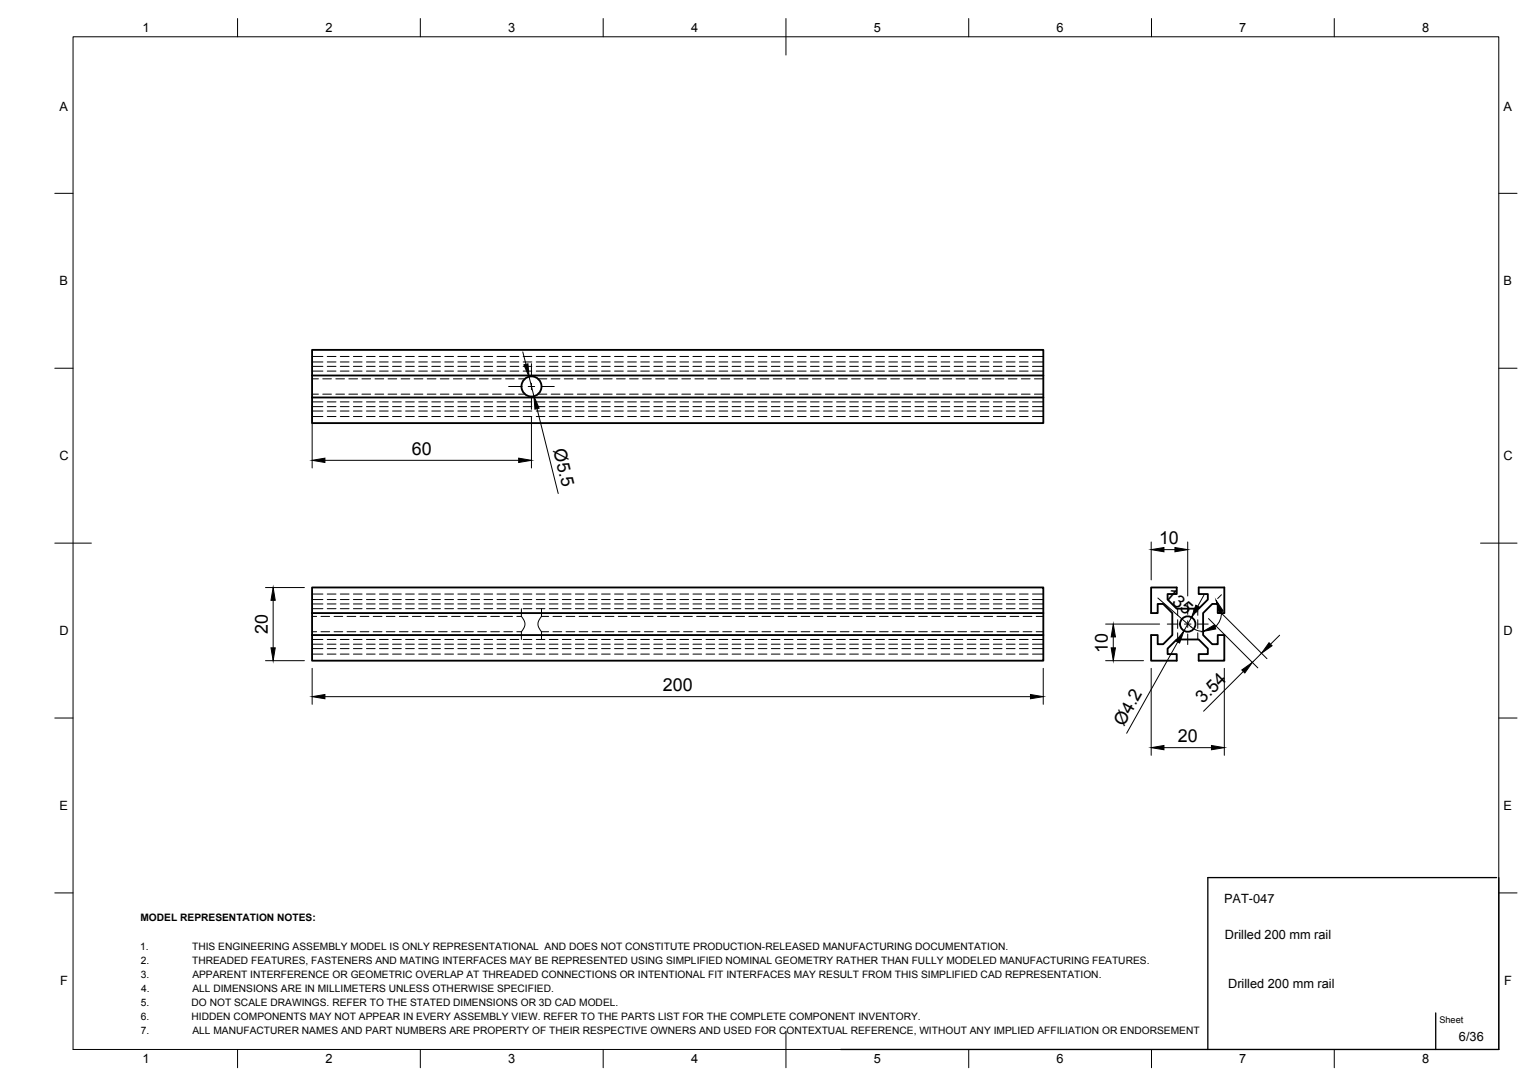
ISO-10303-21;
HEADER;
/* Generated by software containing ST-Developer
 * from STEP Tools, Inc. (www.steptools.com) 
 */

FILE_DESCRIPTION(
/* description */ ('Gravity roller conveyor section'),
/* implementation_level */ '2;1');

FILE_NAME(
/* name */ 'Drilled 200 mm rail.step',
/* time_stamp */ '2026-11-02T07:43:02-08:00',
/* author */ (''),
/* organization */ (''),
/* preprocessor_version */ 'ST-DEVELOPER v20.2',
/* originating_system */ 'Autodesk Translation Framework v15.17.0.0',
/* authorisation */ '');

FILE_SCHEMA (('AUTOMOTIVE_DESIGN { 1 0 10303 214 3 1 1 }'));
ENDSEC;

DATA;
#10=MECHANICAL_DESIGN_GEOMETRIC_PRESENTATION_REPRESENTATION('',(#531),#13821);
#438=B_SPLINE_CURVE_WITH_KNOTS('',3,(#11510,#11511,#11512,#11513,#11514,
#11515,#11516,#11517,#11518,#11519,#11520,#11521,#11522,#11523,#11524,#11525,
#11526,#11527,#11528,#11529,#11530,#11531),.UNSPECIFIED.,.F.,.F.,(4,2,2,
2,2,2,2,2,2,2,4),(0.335938049981195,0.418928967949028,0.501919885916861,
0.586897992939625,0.629387046451008,0.67187609996239,0.714365153473772,
0.756854206985154,0.841832314007919,0.924823231975752,1.00781414994358),
 .UNSPECIFIED.);
#439=B_SPLINE_CURVE_WITH_KNOTS('',3,(#11536,#11537,#11538,#11539,#11540,
#11541,#11542,#11543,#11544,#11545,#11546,#11547),.UNSPECIFIED.,.F.,.F.,
(4,2,2,2,2,4),(0.,0.0424890535113822,0.0849781070227644,0.169956214045529,
0.252947132013362,0.335938049981195),.UNSPECIFIED.);
#440=B_SPLINE_CURVE_WITH_KNOTS('',3,(#11548,#11549,#11550,#11551,#11552,
#11553,#11554,#11555,#11556,#11557,#11558,#11559),.UNSPECIFIED.,.F.,.F.,
(4,2,2,2,2,4),(1.00781414994358,1.09080506791142,1.17379598587925,1.25877409290202,
1.3012631464134,1.34375219992478),.UNSPECIFIED.);
#441=B_SPLINE_CURVE_WITH_KNOTS('',3,(#11562,#11563,#11564,#11565,#11566,
#11567,#11568,#11569,#11570,#11571,#11572,#11573,#11574,#11575,#11576,#11577,
#11578,#11579,#11580,#11581,#11582,#11583,#11584,#11585,#11586,#11587,#11588,
#11589,#11590,#11591,#11592,#11593),.UNSPECIFIED.,.F.,.F.,(4,2,2,2,2,2,
2,2,2,2,2,2,2,2,2,4),(0.,0.0424890535113822,0.0849781070227644,0.169956214045529,
0.252947132013362,0.335938049981195,0.418928967949028,0.501919885916861,
0.586897992939625,0.629387046451008,0.67187609996239,0.714365153473772,
0.756854206985154,0.841832314007919,0.924823231975752,1.00781414994358),
 .UNSPECIFIED.);
#442=B_SPLINE_CURVE_WITH_KNOTS('',3,(#11594,#11595,#11596,#11597,#11598,
#11599,#11600,#11601,#11602,#11603,#11604,#11605),.UNSPECIFIED.,.F.,.F.,
(4,2,2,2,2,4),(1.00781414994358,1.09080506791142,1.17379598587925,1.25877409290202,
1.3012631464134,1.34375219992478),.UNSPECIFIED.);
#463=SHAPE_REPRESENTATION_RELATIONSHIP('SRR','None',#14000,#497);
#497=ADVANCED_BREP_SHAPE_REPRESENTATION('',(#573),#13787);
#531=STYLED_ITEM('',(#14191),#573);
#573=MANIFOLD_SOLID_BREP('Body1',#7629);
#622=FACE_BOUND('',#1499,.T.);
#623=FACE_BOUND('',#1515,.T.);
#624=FACE_BOUND('',#1534,.T.);
#625=FACE_BOUND('',#1549,.T.);
#626=FACE_BOUND('',#1551,.T.);
#754=PLANE('',#8129);
#755=PLANE('',#8130);
#756=PLANE('',#8131);
#757=PLANE('',#8132);
#758=PLANE('',#8133);
#759=PLANE('',#8134);
#760=PLANE('',#8135);
#761=PLANE('',#8136);
#762=PLANE('',#8137);
#763=PLANE('',#8138);
#764=PLANE('',#8139);
#765=PLANE('',#8140);
#766=PLANE('',#8141);
#767=PLANE('',#8142);
#768=PLANE('',#8143);
#769=PLANE('',#8144);
#770=PLANE('',#8145);
#771=PLANE('',#8146);
#772=PLANE('',#8147);
#773=PLANE('',#8148);
#774=PLANE('',#8149);
#775=PLANE('',#8150);
#776=PLANE('',#8151);
#777=PLANE('',#8152);
#778=PLANE('',#8153);
#779=PLANE('',#8154);
#780=PLANE('',#8155);
#781=PLANE('',#8156);
#782=PLANE('',#8157);
#783=PLANE('',#8158);
#784=PLANE('',#8159);
#785=PLANE('',#8160);
#786=PLANE('',#8161);
#787=PLANE('',#8162);
#788=PLANE('',#8163);
#789=PLANE('',#8164);
#790=PLANE('',#8167);
#791=PLANE('',#8168);
#792=PLANE('',#8169);
#793=PLANE('',#8170);
#794=PLANE('',#8171);
#795=PLANE('',#8172);
#796=PLANE('',#8173);
#797=PLANE('',#8174);
#798=PLANE('',#8175);
#799=PLANE('',#8176);
#1066=FACE_OUTER_BOUND('',#1498,.T.);
#1067=FACE_OUTER_BOUND('',#1500,.T.);
#1068=FACE_OUTER_BOUND('',#1501,.T.);
#1069=FACE_OUTER_BOUND('',#1502,.T.);
#1070=FACE_OUTER_BOUND('',#1503,.T.);
#1071=FACE_OUTER_BOUND('',#1504,.T.);
#1072=FACE_OUTER_BOUND('',#1505,.T.);
#1073=FACE_OUTER_BOUND('',#1506,.T.);
#1074=FACE_OUTER_BOUND('',#1507,.T.);
#1075=FACE_OUTER_BOUND('',#1508,.T.);
#1076=FACE_OUTER_BOUND('',#1509,.T.);
#1077=FACE_OUTER_BOUND('',#1510,.T.);
#1078=FACE_OUTER_BOUND('',#1511,.T.);
#1079=FACE_OUTER_BOUND('',#1512,.T.);
#1080=FACE_OUTER_BOUND('',#1513,.T.);
#1081=FACE_OUTER_BOUND('',#1514,.T.);
#1082=FACE_OUTER_BOUND('',#1516,.T.);
#1083=FACE_OUTER_BOUND('',#1517,.T.);
#1084=FACE_OUTER_BOUND('',#1518,.T.);
#1085=FACE_OUTER_BOUND('',#1519,.T.);
#1086=FACE_OUTER_BOUND('',#1520,.T.);
#1087=FACE_OUTER_BOUND('',#1521,.T.);
#1088=FACE_OUTER_BOUND('',#1522,.T.);
#1089=FACE_OUTER_BOUND('',#1523,.T.);
#1090=FACE_OUTER_BOUND('',#1524,.T.);
#1091=FACE_OUTER_BOUND('',#1525,.T.);
#1092=FACE_OUTER_BOUND('',#1526,.T.);
#1093=FACE_OUTER_BOUND('',#1527,.T.);
#1094=FACE_OUTER_BOUND('',#1528,.T.);
#1095=FACE_OUTER_BOUND('',#1529,.T.);
#1096=FACE_OUTER_BOUND('',#1530,.T.);
#1097=FACE_OUTER_BOUND('',#1531,.T.);
#1098=FACE_OUTER_BOUND('',#1532,.T.);
#1099=FACE_OUTER_BOUND('',#1533,.T.);
#1100=FACE_OUTER_BOUND('',#1535,.T.);
#1101=FACE_OUTER_BOUND('',#1536,.T.);
#1102=FACE_OUTER_BOUND('',#1537,.T.);
#1103=FACE_OUTER_BOUND('',#1538,.T.);
#1104=FACE_OUTER_BOUND('',#1539,.T.);
#1105=FACE_OUTER_BOUND('',#1540,.T.);
#1106=FACE_OUTER_BOUND('',#1541,.T.);
#1107=FACE_OUTER_BOUND('',#1542,.T.);
#1108=FACE_OUTER_BOUND('',#1543,.T.);
#1109=FACE_OUTER_BOUND('',#1544,.T.);
#1110=FACE_OUTER_BOUND('',#1545,.T.);
#1111=FACE_OUTER_BOUND('',#1546,.T.);
#1112=FACE_OUTER_BOUND('',#1547,.T.);
#1113=FACE_OUTER_BOUND('',#1548,.T.);
#1114=FACE_OUTER_BOUND('',#1550,.T.);
#1498=EDGE_LOOP('',(#5540,#5541,#5542,#5543,#5544,#5545,#5546,#5547,#5548));
#1499=EDGE_LOOP('',(#5549,#5550));
#1500=EDGE_LOOP('',(#5551,#5552,#5553,#5554,#5555,#5556));
#1501=EDGE_LOOP('',(#5557,#5558,#5559,#5560));
#1502=EDGE_LOOP('',(#5561,#5562,#5563,#5564));
#1503=EDGE_LOOP('',(#5565,#5566,#5567,#5568));
#1504=EDGE_LOOP('',(#5569,#5570,#5571,#5572));
#1505=EDGE_LOOP('',(#5573,#5574,#5575,#5576));
#1506=EDGE_LOOP('',(#5577,#5578,#5579,#5580));
#1507=EDGE_LOOP('',(#5581,#5582,#5583,#5584));
#1508=EDGE_LOOP('',(#5585,#5586,#5587,#5588));
#1509=EDGE_LOOP('',(#5589,#5590,#5591,#5592));
#1510=EDGE_LOOP('',(#5593,#5594,#5595,#5596));
#1511=EDGE_LOOP('',(#5597,#5598,#5599,#5600));
#1512=EDGE_LOOP('',(#5601,#5602,#5603,#5604));
#1513=EDGE_LOOP('',(#5605,#5606,#5607,#5608));
#1514=EDGE_LOOP('',(#5609,#5610,#5611,#5612));
#1515=EDGE_LOOP('',(#5613));
#1516=EDGE_LOOP('',(#5614,#5615,#5616,#5617));
#1517=EDGE_LOOP('',(#5618,#5619,#5620,#5621));
#1518=EDGE_LOOP('',(#5622,#5623,#5624,#5625));
#1519=EDGE_LOOP('',(#5626,#5627,#5628,#5629));
#1520=EDGE_LOOP('',(#5630,#5631,#5632,#5633));
#1521=EDGE_LOOP('',(#5634,#5635,#5636,#5637));
#1522=EDGE_LOOP('',(#5638,#5639,#5640,#5641));
#1523=EDGE_LOOP('',(#5642,#5643,#5644,#5645));
#1524=EDGE_LOOP('',(#5646,#5647,#5648,#5649));
#1525=EDGE_LOOP('',(#5650,#5651,#5652,#5653));
#1526=EDGE_LOOP('',(#5654,#5655,#5656,#5657));
#1527=EDGE_LOOP('',(#5658,#5659,#5660,#5661));
#1528=EDGE_LOOP('',(#5662,#5663,#5664,#5665));
#1529=EDGE_LOOP('',(#5666,#5667,#5668,#5669));
#1530=EDGE_LOOP('',(#5670,#5671,#5672,#5673));
#1531=EDGE_LOOP('',(#5674,#5675,#5676,#5677));
#1532=EDGE_LOOP('',(#5678,#5679,#5680,#5681));
#1533=EDGE_LOOP('',(#5682,#5683,#5684,#5685));
#1534=EDGE_LOOP('',(#5686));
#1535=EDGE_LOOP('',(#5687,#5688,#5689,#5690));
#1536=EDGE_LOOP('',(#5691,#5692,#5693,#5694));
#1537=EDGE_LOOP('',(#5695,#5696,#5697,#5698));
#1538=EDGE_LOOP('',(#5699,#5700,#5701,#5702));
#1539=EDGE_LOOP('',(#5703,#5704,#5705,#5706,#5707));
#1540=EDGE_LOOP('',(#5708,#5709,#5710,#5711));
#1541=EDGE_LOOP('',(#5712,#5713,#5714,#5715));
#1542=EDGE_LOOP('',(#5716,#5717,#5718,#5719));
#1543=EDGE_LOOP('',(#5720,#5721,#5722,#5723));
#1544=EDGE_LOOP('',(#5724,#5725,#5726,#5727));
#1545=EDGE_LOOP('',(#5728,#5729,#5730,#5731));
#1546=EDGE_LOOP('',(#5732,#5733,#5734,#5735));
#1547=EDGE_LOOP('',(#5736,#5737,#5738,#5739));
#1548=EDGE_LOOP('',(#5740,#5741,#5742,#5743,#5744,#5745,#5746,#5747,#5748,
#5749,#5750,#5751,#5752,#5753,#5754,#5755,#5756,#5757,#5758,#5759,#5760,
#5761,#5762,#5763,#5764,#5765,#5766,#5767,#5768,#5769,#5770,#5771,#5772,
#5773,#5774,#5775,#5776,#5777,#5778,#5779,#5780,#5781,#5782,#5783));
#1549=EDGE_LOOP('',(#5784));
#1550=EDGE_LOOP('',(#5785,#5786,#5787,#5788,#5789,#5790,#5791,#5792,#5793,
#5794,#5795,#5796,#5797,#5798,#5799,#5800,#5801,#5802,#5803,#5804,#5805,
#5806,#5807,#5808,#5809,#5810,#5811,#5812,#5813,#5814,#5815,#5816,#5817,
#5818,#5819,#5820,#5821,#5822,#5823,#5824,#5825,#5826,#5827,#5828));
#1551=EDGE_LOOP('',(#5829));
#2090=LINE('',#11508,#2808);
#2091=LINE('',#11533,#2809);
#2092=LINE('',#11609,#2810);
#2093=LINE('',#11613,#2811);
#2094=LINE('',#11615,#2812);
#2095=LINE('',#11617,#2813);
#2096=LINE('',#11618,#2814);
#2097=LINE('',#11621,#2815);
#2098=LINE('',#11623,#2816);
#2099=LINE('',#11624,#2817);
#2100=LINE('',#11627,#2818);
#2101=LINE('',#11629,#2819);
#2102=LINE('',#11630,#2820);
#2103=LINE('',#11633,#2821);
#2104=LINE('',#11635,#2822);
#2105=LINE('',#11636,#2823);
#2106=LINE('',#11639,#2824);
#2107=LINE('',#11641,#2825);
#2108=LINE('',#11642,#2826);
#2109=LINE('',#11645,#2827);
#2110=LINE('',#11647,#2828);
#2111=LINE('',#11648,#2829);
#2112=LINE('',#11651,#2830);
#2113=LINE('',#11653,#2831);
#2114=LINE('',#11654,#2832);
#2115=LINE('',#11657,#2833);
#2116=LINE('',#11659,#2834);
#2117=LINE('',#11660,#2835);
#2118=LINE('',#11663,#2836);
#2119=LINE('',#11665,#2837);
#2120=LINE('',#11666,#2838);
#2121=LINE('',#11670,#2839);
#2122=LINE('',#11672,#2840);
#2123=LINE('',#11674,#2841);
#2124=LINE('',#11675,#2842);
#2125=LINE('',#11678,#2843);
#2126=LINE('',#11680,#2844);
#2127=LINE('',#11681,#2845);
#2128=LINE('',#11684,#2846);
#2129=LINE('',#11686,#2847);
#2130=LINE('',#11687,#2848);
#2131=LINE('',#11690,#2849);
#2132=LINE('',#11692,#2850);
#2133=LINE('',#11693,#2851);
#2134=LINE('',#11696,#2852);
#2135=LINE('',#11698,#2853);
#2136=LINE('',#11699,#2854);
#2137=LINE('',#11702,#2855);
#2138=LINE('',#11704,#2856);
#2139=LINE('',#11705,#2857);
#2140=LINE('',#11708,#2858);
#2141=LINE('',#11710,#2859);
#2142=LINE('',#11711,#2860);
#2143=LINE('',#11714,#2861);
#2144=LINE('',#11716,#2862);
#2145=LINE('',#11717,#2863);
#2146=LINE('',#11720,#2864);
#2147=LINE('',#11722,#2865);
#2148=LINE('',#11723,#2866);
#2149=LINE('',#11727,#2867);
#2150=LINE('',#11729,#2868);
#2151=LINE('',#11731,#2869);
#2152=LINE('',#11732,#2870);
#2153=LINE('',#11735,#2871);
#2154=LINE('',#11737,#2872);
#2155=LINE('',#11738,#2873);
#2156=LINE('',#11741,#2874);
#2157=LINE('',#11743,#2875);
#2158=LINE('',#11744,#2876);
#2159=LINE('',#11747,#2877);
#2160=LINE('',#11749,#2878);
#2161=LINE('',#11750,#2879);
#2162=LINE('',#11753,#2880);
#2163=LINE('',#11755,#2881);
#2164=LINE('',#11756,#2882);
#2165=LINE('',#11759,#2883);
#2166=LINE('',#11761,#2884);
#2167=LINE('',#11762,#2885);
#2168=LINE('',#11765,#2886);
#2169=LINE('',#11767,#2887);
#2170=LINE('',#11768,#2888);
#2171=LINE('',#11771,#2889);
#2172=LINE('',#11773,#2890);
#2173=LINE('',#11774,#2891);
#2174=LINE('',#11777,#2892);
#2175=LINE('',#11779,#2893);
#2176=LINE('',#11780,#2894);
#2177=LINE('',#11784,#2895);
#2178=LINE('',#11786,#2896);
#2179=LINE('',#11788,#2897);
#2180=LINE('',#11789,#2898);
#2181=LINE('',#11792,#2899);
#2182=LINE('',#11794,#2900);
#2183=LINE('',#11795,#2901);
#2184=LINE('',#11798,#2902);
#2185=LINE('',#11800,#2903);
#2186=LINE('',#11801,#2904);
#2187=LINE('',#11804,#2905);
#2188=LINE('',#11806,#2906);
#2189=LINE('',#11807,#2907);
#2190=LINE('',#11810,#2908);
#2191=LINE('',#11812,#2909);
#2192=LINE('',#11813,#2910);
#2193=LINE('',#11816,#2911);
#2194=LINE('',#11818,#2912);
#2195=LINE('',#11819,#2913);
#2196=LINE('',#11822,#2914);
#2197=LINE('',#11824,#2915);
#2198=LINE('',#11825,#2916);
#2199=LINE('',#11828,#2917);
#2200=LINE('',#11830,#2918);
#2201=LINE('',#11831,#2919);
#2202=LINE('',#11834,#2920);
#2203=LINE('',#11836,#2921);
#2204=LINE('',#11837,#2922);
#2205=LINE('',#11840,#2923);
#2206=LINE('',#11844,#2924);
#2207=LINE('',#11846,#2925);
#2208=LINE('',#11847,#2926);
#2209=LINE('',#11850,#2927);
#2210=LINE('',#11852,#2928);
#2211=LINE('',#11853,#2929);
#2212=LINE('',#11855,#2930);
#2213=LINE('',#11856,#2931);
#2214=LINE('',#11859,#2932);
#2215=LINE('',#11861,#2933);
#2216=LINE('',#11862,#2934);
#2217=LINE('',#11864,#2935);
#2218=LINE('',#11865,#2936);
#2219=LINE('',#11868,#2937);
#2220=LINE('',#11870,#2938);
#2221=LINE('',#11871,#2939);
#2222=LINE('',#11873,#2940);
#2223=LINE('',#11874,#2941);
#2224=LINE('',#11876,#2942);
#2225=LINE('',#11877,#2943);
#2808=VECTOR('',#9125,0.275);
#2809=VECTOR('',#9126,0.275);
#2810=VECTOR('',#9133,0.21);
#2811=VECTOR('',#9136,1.);
#2812=VECTOR('',#9137,1.);
#2813=VECTOR('',#9138,1.);
#2814=VECTOR('',#9139,1.);
#2815=VECTOR('',#9142,1.);
#2816=VECTOR('',#9143,1.);
#2817=VECTOR('',#9144,1.);
#2818=VECTOR('',#9147,1.);
#2819=VECTOR('',#9148,1.);
#2820=VECTOR('',#9149,1.);
#2821=VECTOR('',#9152,1.);
#2822=VECTOR('',#9153,1.);
#2823=VECTOR('',#9154,1.);
#2824=VECTOR('',#9157,1.);
#2825=VECTOR('',#9158,1.);
#2826=VECTOR('',#9159,1.);
#2827=VECTOR('',#9162,1.);
#2828=VECTOR('',#9163,1.);
#2829=VECTOR('',#9164,1.);
#2830=VECTOR('',#9167,1.);
#2831=VECTOR('',#9168,1.);
#2832=VECTOR('',#9169,1.);
#2833=VECTOR('',#9172,1.);
#2834=VECTOR('',#9173,1.);
#2835=VECTOR('',#9174,1.);
#2836=VECTOR('',#9177,1.);
#2837=VECTOR('',#9178,1.);
#2838=VECTOR('',#9179,1.);
#2839=VECTOR('',#9182,1.);
#2840=VECTOR('',#9183,1.);
#2841=VECTOR('',#9184,1.);
#2842=VECTOR('',#9185,1.);
#2843=VECTOR('',#9188,1.);
#2844=VECTOR('',#9189,1.);
#2845=VECTOR('',#9190,1.);
#2846=VECTOR('',#9193,1.);
#2847=VECTOR('',#9194,1.);
#2848=VECTOR('',#9195,1.);
#2849=VECTOR('',#9198,1.);
#2850=VECTOR('',#9199,1.);
#2851=VECTOR('',#9200,1.);
#2852=VECTOR('',#9203,1.);
#2853=VECTOR('',#9204,1.);
#2854=VECTOR('',#9205,1.);
#2855=VECTOR('',#9208,1.);
#2856=VECTOR('',#9209,1.);
#2857=VECTOR('',#9210,1.);
#2858=VECTOR('',#9213,1.);
#2859=VECTOR('',#9214,1.);
#2860=VECTOR('',#9215,1.);
#2861=VECTOR('',#9218,1.);
#2862=VECTOR('',#9219,1.);
#2863=VECTOR('',#9220,1.);
#2864=VECTOR('',#9223,1.);
#2865=VECTOR('',#9224,1.);
#2866=VECTOR('',#9225,1.);
#2867=VECTOR('',#9228,1.);
#2868=VECTOR('',#9229,1.);
#2869=VECTOR('',#9230,1.);
#2870=VECTOR('',#9231,1.);
#2871=VECTOR('',#9234,1.);
#2872=VECTOR('',#9235,1.);
#2873=VECTOR('',#9236,1.);
#2874=VECTOR('',#9239,1.);
#2875=VECTOR('',#9240,1.);
#2876=VECTOR('',#9241,1.);
#2877=VECTOR('',#9244,1.);
#2878=VECTOR('',#9245,1.);
#2879=VECTOR('',#9246,1.);
#2880=VECTOR('',#9249,1.);
#2881=VECTOR('',#9250,1.);
#2882=VECTOR('',#9251,1.);
#2883=VECTOR('',#9254,1.);
#2884=VECTOR('',#9255,1.);
#2885=VECTOR('',#9256,1.);
#2886=VECTOR('',#9259,1.);
#2887=VECTOR('',#9260,1.);
#2888=VECTOR('',#9261,1.);
#2889=VECTOR('',#9264,1.);
#2890=VECTOR('',#9265,1.);
#2891=VECTOR('',#9266,1.);
#2892=VECTOR('',#9269,1.);
#2893=VECTOR('',#9270,1.);
#2894=VECTOR('',#9271,1.);
#2895=VECTOR('',#9274,1.);
#2896=VECTOR('',#9275,1.);
#2897=VECTOR('',#9276,1.);
#2898=VECTOR('',#9277,1.);
#2899=VECTOR('',#9280,1.);
#2900=VECTOR('',#9281,1.);
#2901=VECTOR('',#9282,1.);
#2902=VECTOR('',#9285,1.);
#2903=VECTOR('',#9286,1.);
#2904=VECTOR('',#9287,1.);
#2905=VECTOR('',#9290,1.);
#2906=VECTOR('',#9291,1.);
#2907=VECTOR('',#9292,1.);
#2908=VECTOR('',#9295,1.);
#2909=VECTOR('',#9296,1.);
#2910=VECTOR('',#9297,1.);
#2911=VECTOR('',#9300,1.);
#2912=VECTOR('',#9301,1.);
#2913=VECTOR('',#9302,1.);
#2914=VECTOR('',#9305,1.);
#2915=VECTOR('',#9306,1.);
#2916=VECTOR('',#9307,1.);
#2917=VECTOR('',#9310,1.);
#2918=VECTOR('',#9311,1.);
#2919=VECTOR('',#9312,1.);
#2920=VECTOR('',#9315,1.);
#2921=VECTOR('',#9316,1.);
#2922=VECTOR('',#9317,1.);
#2923=VECTOR('',#9320,0.21);
#2924=VECTOR('',#9325,1.);
#2925=VECTOR('',#9326,1.);
#2926=VECTOR('',#9327,1.);
#2927=VECTOR('',#9330,1.);
#2928=VECTOR('',#9331,1.);
#2929=VECTOR('',#9332,1.);
#2930=VECTOR('',#9335,1.);
#2931=VECTOR('',#9336,1.);
#2932=VECTOR('',#9339,1.);
#2933=VECTOR('',#9340,1.);
#2934=VECTOR('',#9341,1.);
#2935=VECTOR('',#9344,1.);
#2936=VECTOR('',#9345,1.);
#2937=VECTOR('',#9348,1.);
#2938=VECTOR('',#9349,1.);
#2939=VECTOR('',#9350,1.);
#2940=VECTOR('',#9353,1.);
#2941=VECTOR('',#9354,1.);
#2942=VECTOR('',#9357,1.);
#2943=VECTOR('',#9358,1.);
#3386=CIRCLE('',#8125,0.275);
#3387=CIRCLE('',#8126,0.275);
#3388=CIRCLE('',#8128,0.21);
#3389=CIRCLE('',#8166,0.21);
#3703=VERTEX_POINT('',#11505);
#3704=VERTEX_POINT('',#11507);
#3705=VERTEX_POINT('',#11509);
#3706=VERTEX_POINT('',#11532);
#3707=VERTEX_POINT('',#11535);
#3708=VERTEX_POINT('',#11560);
#3709=VERTEX_POINT('',#11561);
#3710=VERTEX_POINT('',#11607);
#3711=VERTEX_POINT('',#11611);
#3712=VERTEX_POINT('',#11612);
#3713=VERTEX_POINT('',#11614);
#3714=VERTEX_POINT('',#11616);
#3715=VERTEX_POINT('',#11620);
#3716=VERTEX_POINT('',#11622);
#3717=VERTEX_POINT('',#11626);
#3718=VERTEX_POINT('',#11628);
#3719=VERTEX_POINT('',#11632);
#3720=VERTEX_POINT('',#11634);
#3721=VERTEX_POINT('',#11638);
#3722=VERTEX_POINT('',#11640);
#3723=VERTEX_POINT('',#11644);
#3724=VERTEX_POINT('',#11646);
#3725=VERTEX_POINT('',#11650);
#3726=VERTEX_POINT('',#11652);
#3727=VERTEX_POINT('',#11656);
#3728=VERTEX_POINT('',#11658);
#3729=VERTEX_POINT('',#11662);
#3730=VERTEX_POINT('',#11664);
#3731=VERTEX_POINT('',#11668);
#3732=VERTEX_POINT('',#11669);
#3733=VERTEX_POINT('',#11671);
#3734=VERTEX_POINT('',#11673);
#3735=VERTEX_POINT('',#11677);
#3736=VERTEX_POINT('',#11679);
#3737=VERTEX_POINT('',#11683);
#3738=VERTEX_POINT('',#11685);
#3739=VERTEX_POINT('',#11689);
#3740=VERTEX_POINT('',#11691);
#3741=VERTEX_POINT('',#11695);
#3742=VERTEX_POINT('',#11697);
#3743=VERTEX_POINT('',#11701);
#3744=VERTEX_POINT('',#11703);
#3745=VERTEX_POINT('',#11707);
#3746=VERTEX_POINT('',#11709);
#3747=VERTEX_POINT('',#11713);
#3748=VERTEX_POINT('',#11715);
#3749=VERTEX_POINT('',#11719);
#3750=VERTEX_POINT('',#11721);
#3751=VERTEX_POINT('',#11725);
#3752=VERTEX_POINT('',#11726);
#3753=VERTEX_POINT('',#11728);
#3754=VERTEX_POINT('',#11730);
#3755=VERTEX_POINT('',#11734);
#3756=VERTEX_POINT('',#11736);
#3757=VERTEX_POINT('',#11740);
#3758=VERTEX_POINT('',#11742);
#3759=VERTEX_POINT('',#11746);
#3760=VERTEX_POINT('',#11748);
#3761=VERTEX_POINT('',#11752);
#3762=VERTEX_POINT('',#11754);
#3763=VERTEX_POINT('',#11758);
#3764=VERTEX_POINT('',#11760);
#3765=VERTEX_POINT('',#11764);
#3766=VERTEX_POINT('',#11766);
#3767=VERTEX_POINT('',#11770);
#3768=VERTEX_POINT('',#11772);
#3769=VERTEX_POINT('',#11776);
#3770=VERTEX_POINT('',#11778);
#3771=VERTEX_POINT('',#11782);
#3772=VERTEX_POINT('',#11783);
#3773=VERTEX_POINT('',#11785);
#3774=VERTEX_POINT('',#11787);
#3775=VERTEX_POINT('',#11791);
#3776=VERTEX_POINT('',#11793);
#3777=VERTEX_POINT('',#11797);
#3778=VERTEX_POINT('',#11799);
#3779=VERTEX_POINT('',#11803);
#3780=VERTEX_POINT('',#11805);
#3781=VERTEX_POINT('',#11809);
#3782=VERTEX_POINT('',#11811);
#3783=VERTEX_POINT('',#11815);
#3784=VERTEX_POINT('',#11817);
#3785=VERTEX_POINT('',#11821);
#3786=VERTEX_POINT('',#11823);
#3787=VERTEX_POINT('',#11827);
#3788=VERTEX_POINT('',#11829);
#3789=VERTEX_POINT('',#11833);
#3790=VERTEX_POINT('',#11835);
#3791=VERTEX_POINT('',#11839);
#3792=VERTEX_POINT('',#11843);
#3793=VERTEX_POINT('',#11845);
#3794=VERTEX_POINT('',#11849);
#3795=VERTEX_POINT('',#11851);
#3796=VERTEX_POINT('',#11858);
#3797=VERTEX_POINT('',#11860);
#3798=VERTEX_POINT('',#11867);
#3799=VERTEX_POINT('',#11869);
#4407=EDGE_CURVE('',#3703,#3703,#3386,.T.);
#4408=EDGE_CURVE('',#3703,#3704,#2090,.T.);
#4409=EDGE_CURVE('',#3705,#3704,#438,.T.);
#4410=EDGE_CURVE('',#3705,#3706,#2091,.T.);
#4411=EDGE_CURVE('',#3706,#3706,#3387,.T.);
#4412=EDGE_CURVE('',#3707,#3705,#439,.T.);
#4413=EDGE_CURVE('',#3704,#3707,#440,.T.);
#4414=EDGE_CURVE('',#3708,#3709,#441,.T.);
#4415=EDGE_CURVE('',#3709,#3708,#442,.T.);
#4416=EDGE_CURVE('',#3710,#3710,#3388,.T.);
#4417=EDGE_CURVE('',#3710,#3705,#2092,.T.);
#4418=EDGE_CURVE('',#3711,#3712,#2093,.T.);
#4419=EDGE_CURVE('',#3711,#3713,#2094,.T.);
#4420=EDGE_CURVE('',#3714,#3713,#2095,.T.);
#4421=EDGE_CURVE('',#3712,#3714,#2096,.T.);
#4422=EDGE_CURVE('',#3715,#3711,#2097,.T.);
#4423=EDGE_CURVE('',#3715,#3716,#2098,.T.);
#4424=EDGE_CURVE('',#3713,#3716,#2099,.T.);
#4425=EDGE_CURVE('',#3717,#3715,#2100,.T.);
#4426=EDGE_CURVE('',#3717,#3718,#2101,.T.);
#4427=EDGE_CURVE('',#3716,#3718,#2102,.T.);
#4428=EDGE_CURVE('',#3719,#3717,#2103,.T.);
#4429=EDGE_CURVE('',#3719,#3720,#2104,.T.);
#4430=EDGE_CURVE('',#3718,#3720,#2105,.T.);
#4431=EDGE_CURVE('',#3721,#3719,#2106,.T.);
#4432=EDGE_CURVE('',#3721,#3722,#2107,.T.);
#4433=EDGE_CURVE('',#3720,#3722,#2108,.T.);
#4434=EDGE_CURVE('',#3723,#3721,#2109,.T.);
#4435=EDGE_CURVE('',#3723,#3724,#2110,.T.);
#4436=EDGE_CURVE('',#3722,#3724,#2111,.T.);
#4437=EDGE_CURVE('',#3725,#3723,#2112,.T.);
#4438=EDGE_CURVE('',#3725,#3726,#2113,.T.);
#4439=EDGE_CURVE('',#3724,#3726,#2114,.T.);
#4440=EDGE_CURVE('',#3727,#3725,#2115,.T.);
#4441=EDGE_CURVE('',#3727,#3728,#2116,.T.);
#4442=EDGE_CURVE('',#3726,#3728,#2117,.T.);
#4443=EDGE_CURVE('',#3729,#3727,#2118,.T.);
#4444=EDGE_CURVE('',#3730,#3729,#2119,.T.);
#4445=EDGE_CURVE('',#3728,#3730,#2120,.T.);
#4446=EDGE_CURVE('',#3731,#3732,#2121,.T.);
#4447=EDGE_CURVE('',#3731,#3733,#2122,.T.);
#4448=EDGE_CURVE('',#3734,#3733,#2123,.T.);
#4449=EDGE_CURVE('',#3732,#3734,#2124,.T.);
#4450=EDGE_CURVE('',#3735,#3731,#2125,.T.);
#4451=EDGE_CURVE('',#3735,#3736,#2126,.T.);
#4452=EDGE_CURVE('',#3733,#3736,#2127,.T.);
#4453=EDGE_CURVE('',#3737,#3735,#2128,.T.);
#4454=EDGE_CURVE('',#3737,#3738,#2129,.T.);
#4455=EDGE_CURVE('',#3736,#3738,#2130,.T.);
#4456=EDGE_CURVE('',#3739,#3737,#2131,.T.);
#4457=EDGE_CURVE('',#3739,#3740,#2132,.T.);
#4458=EDGE_CURVE('',#3738,#3740,#2133,.T.);
#4459=EDGE_CURVE('',#3741,#3739,#2134,.T.);
#4460=EDGE_CURVE('',#3741,#3742,#2135,.T.);
#4461=EDGE_CURVE('',#3740,#3742,#2136,.T.);
#4462=EDGE_CURVE('',#3743,#3741,#2137,.T.);
#4463=EDGE_CURVE('',#3743,#3744,#2138,.T.);
#4464=EDGE_CURVE('',#3742,#3744,#2139,.T.);
#4465=EDGE_CURVE('',#3745,#3743,#2140,.T.);
#4466=EDGE_CURVE('',#3745,#3746,#2141,.T.);
#4467=EDGE_CURVE('',#3744,#3746,#2142,.T.);
#4468=EDGE_CURVE('',#3747,#3745,#2143,.T.);
#4469=EDGE_CURVE('',#3747,#3748,#2144,.T.);
#4470=EDGE_CURVE('',#3746,#3748,#2145,.T.);
#4471=EDGE_CURVE('',#3749,#3747,#2146,.T.);
#4472=EDGE_CURVE('',#3750,#3749,#2147,.T.);
#4473=EDGE_CURVE('',#3748,#3750,#2148,.T.);
#4474=EDGE_CURVE('',#3751,#3752,#2149,.T.);
#4475=EDGE_CURVE('',#3751,#3753,#2150,.T.);
#4476=EDGE_CURVE('',#3754,#3753,#2151,.T.);
#4477=EDGE_CURVE('',#3752,#3754,#2152,.T.);
#4478=EDGE_CURVE('',#3755,#3751,#2153,.T.);
#4479=EDGE_CURVE('',#3755,#3756,#2154,.T.);
#4480=EDGE_CURVE('',#3753,#3756,#2155,.T.);
#4481=EDGE_CURVE('',#3757,#3755,#2156,.T.);
#4482=EDGE_CURVE('',#3757,#3758,#2157,.T.);
#4483=EDGE_CURVE('',#3756,#3758,#2158,.T.);
#4484=EDGE_CURVE('',#3759,#3757,#2159,.T.);
#4485=EDGE_CURVE('',#3759,#3760,#2160,.T.);
#4486=EDGE_CURVE('',#3758,#3760,#2161,.T.);
#4487=EDGE_CURVE('',#3761,#3759,#2162,.T.);
#4488=EDGE_CURVE('',#3761,#3762,#2163,.T.);
#4489=EDGE_CURVE('',#3760,#3762,#2164,.T.);
#4490=EDGE_CURVE('',#3763,#3761,#2165,.T.);
#4491=EDGE_CURVE('',#3763,#3764,#2166,.T.);
#4492=EDGE_CURVE('',#3762,#3764,#2167,.T.);
#4493=EDGE_CURVE('',#3765,#3763,#2168,.T.);
#4494=EDGE_CURVE('',#3765,#3766,#2169,.T.);
#4495=EDGE_CURVE('',#3764,#3766,#2170,.T.);
#4496=EDGE_CURVE('',#3767,#3765,#2171,.T.);
#4497=EDGE_CURVE('',#3767,#3768,#2172,.T.);
#4498=EDGE_CURVE('',#3766,#3768,#2173,.T.);
#4499=EDGE_CURVE('',#3769,#3767,#2174,.T.);
#4500=EDGE_CURVE('',#3770,#3769,#2175,.T.);
#4501=EDGE_CURVE('',#3768,#3770,#2176,.T.);
#4502=EDGE_CURVE('',#3771,#3772,#2177,.T.);
#4503=EDGE_CURVE('',#3771,#3773,#2178,.T.);
#4504=EDGE_CURVE('',#3774,#3773,#2179,.T.);
#4505=EDGE_CURVE('',#3772,#3774,#2180,.T.);
#4506=EDGE_CURVE('',#3775,#3771,#2181,.T.);
#4507=EDGE_CURVE('',#3775,#3776,#2182,.T.);
#4508=EDGE_CURVE('',#3773,#3776,#2183,.T.);
#4509=EDGE_CURVE('',#3777,#3775,#2184,.T.);
#4510=EDGE_CURVE('',#3777,#3778,#2185,.T.);
#4511=EDGE_CURVE('',#3776,#3778,#2186,.T.);
#4512=EDGE_CURVE('',#3779,#3777,#2187,.T.);
#4513=EDGE_CURVE('',#3779,#3780,#2188,.T.);
#4514=EDGE_CURVE('',#3778,#3780,#2189,.T.);
#4515=EDGE_CURVE('',#3781,#3779,#2190,.T.);
#4516=EDGE_CURVE('',#3781,#3782,#2191,.T.);
#4517=EDGE_CURVE('',#3780,#3782,#2192,.T.);
#4518=EDGE_CURVE('',#3783,#3781,#2193,.T.);
#4519=EDGE_CURVE('',#3783,#3784,#2194,.T.);
#4520=EDGE_CURVE('',#3782,#3784,#2195,.T.);
#4521=EDGE_CURVE('',#3785,#3783,#2196,.T.);
#4522=EDGE_CURVE('',#3785,#3786,#2197,.T.);
#4523=EDGE_CURVE('',#3784,#3786,#2198,.T.);
#4524=EDGE_CURVE('',#3787,#3785,#2199,.T.);
#4525=EDGE_CURVE('',#3787,#3788,#2200,.T.);
#4526=EDGE_CURVE('',#3786,#3788,#2201,.T.);
#4527=EDGE_CURVE('',#3789,#3787,#2202,.T.);
#4528=EDGE_CURVE('',#3790,#3789,#2203,.T.);
#4529=EDGE_CURVE('',#3788,#3790,#2204,.T.);
#4530=EDGE_CURVE('',#3709,#3791,#2205,.T.);
#4531=EDGE_CURVE('',#3791,#3791,#3389,.T.);
#4532=EDGE_CURVE('',#3729,#3792,#2206,.T.);
#4533=EDGE_CURVE('',#3792,#3793,#2207,.T.);
#4534=EDGE_CURVE('',#3730,#3793,#2208,.T.);
#4535=EDGE_CURVE('',#3794,#3714,#2209,.T.);
#4536=EDGE_CURVE('',#3795,#3794,#2210,.T.);
#4537=EDGE_CURVE('',#3795,#3712,#2211,.T.);
#4538=EDGE_CURVE('',#3749,#3795,#2212,.T.);
#4539=EDGE_CURVE('',#3750,#3794,#2213,.T.);
#4540=EDGE_CURVE('',#3796,#3734,#2214,.T.);
#4541=EDGE_CURVE('',#3797,#3796,#2215,.T.);
#4542=EDGE_CURVE('',#3797,#3732,#2216,.T.);
#4543=EDGE_CURVE('',#3769,#3797,#2217,.T.);
#4544=EDGE_CURVE('',#3770,#3796,#2218,.T.);
#4545=EDGE_CURVE('',#3798,#3754,#2219,.T.);
#4546=EDGE_CURVE('',#3799,#3798,#2220,.T.);
#4547=EDGE_CURVE('',#3799,#3752,#2221,.T.);
#4548=EDGE_CURVE('',#3789,#3799,#2222,.T.);
#4549=EDGE_CURVE('',#3790,#3798,#2223,.T.);
#4550=EDGE_CURVE('',#3793,#3774,#2224,.T.);
#4551=EDGE_CURVE('',#3792,#3772,#2225,.T.);
#5540=ORIENTED_EDGE('',*,*,#4407,.F.);
#5541=ORIENTED_EDGE('',*,*,#4408,.T.);
#5542=ORIENTED_EDGE('',*,*,#4409,.F.);
#5543=ORIENTED_EDGE('',*,*,#4410,.T.);
#5544=ORIENTED_EDGE('',*,*,#4411,.F.);
#5545=ORIENTED_EDGE('',*,*,#4410,.F.);
#5546=ORIENTED_EDGE('',*,*,#4412,.F.);
#5547=ORIENTED_EDGE('',*,*,#4413,.F.);
#5548=ORIENTED_EDGE('',*,*,#4408,.F.);
#5549=ORIENTED_EDGE('',*,*,#4414,.F.);
#5550=ORIENTED_EDGE('',*,*,#4415,.F.);
#5551=ORIENTED_EDGE('',*,*,#4416,.F.);
#5552=ORIENTED_EDGE('',*,*,#4417,.T.);
#5553=ORIENTED_EDGE('',*,*,#4409,.T.);
#5554=ORIENTED_EDGE('',*,*,#4413,.T.);
#5555=ORIENTED_EDGE('',*,*,#4412,.T.);
#5556=ORIENTED_EDGE('',*,*,#4417,.F.);
#5557=ORIENTED_EDGE('',*,*,#4418,.F.);
#5558=ORIENTED_EDGE('',*,*,#4419,.T.);
#5559=ORIENTED_EDGE('',*,*,#4420,.F.);
#5560=ORIENTED_EDGE('',*,*,#4421,.F.);
#5561=ORIENTED_EDGE('',*,*,#4422,.F.);
#5562=ORIENTED_EDGE('',*,*,#4423,.T.);
#5563=ORIENTED_EDGE('',*,*,#4424,.F.);
#5564=ORIENTED_EDGE('',*,*,#4419,.F.);
#5565=ORIENTED_EDGE('',*,*,#4425,.F.);
#5566=ORIENTED_EDGE('',*,*,#4426,.T.);
#5567=ORIENTED_EDGE('',*,*,#4427,.F.);
#5568=ORIENTED_EDGE('',*,*,#4423,.F.);
#5569=ORIENTED_EDGE('',*,*,#4428,.F.);
#5570=ORIENTED_EDGE('',*,*,#4429,.T.);
#5571=ORIENTED_EDGE('',*,*,#4430,.F.);
#5572=ORIENTED_EDGE('',*,*,#4426,.F.);
#5573=ORIENTED_EDGE('',*,*,#4431,.F.);
#5574=ORIENTED_EDGE('',*,*,#4432,.T.);
#5575=ORIENTED_EDGE('',*,*,#4433,.F.);
#5576=ORIENTED_EDGE('',*,*,#4429,.F.);
#5577=ORIENTED_EDGE('',*,*,#4434,.F.);
#5578=ORIENTED_EDGE('',*,*,#4435,.T.);
#5579=ORIENTED_EDGE('',*,*,#4436,.F.);
#5580=ORIENTED_EDGE('',*,*,#4432,.F.);
#5581=ORIENTED_EDGE('',*,*,#4437,.F.);
#5582=ORIENTED_EDGE('',*,*,#4438,.T.);
#5583=ORIENTED_EDGE('',*,*,#4439,.F.);
#5584=ORIENTED_EDGE('',*,*,#4435,.F.);
#5585=ORIENTED_EDGE('',*,*,#4440,.F.);
#5586=ORIENTED_EDGE('',*,*,#4441,.T.);
#5587=ORIENTED_EDGE('',*,*,#4442,.F.);
#5588=ORIENTED_EDGE('',*,*,#4438,.F.);
#5589=ORIENTED_EDGE('',*,*,#4443,.F.);
#5590=ORIENTED_EDGE('',*,*,#4444,.F.);
#5591=ORIENTED_EDGE('',*,*,#4445,.F.);
#5592=ORIENTED_EDGE('',*,*,#4441,.F.);
#5593=ORIENTED_EDGE('',*,*,#4446,.F.);
#5594=ORIENTED_EDGE('',*,*,#4447,.T.);
#5595=ORIENTED_EDGE('',*,*,#4448,.F.);
#5596=ORIENTED_EDGE('',*,*,#4449,.F.);
#5597=ORIENTED_EDGE('',*,*,#4450,.F.);
#5598=ORIENTED_EDGE('',*,*,#4451,.T.);
#5599=ORIENTED_EDGE('',*,*,#4452,.F.);
#5600=ORIENTED_EDGE('',*,*,#4447,.F.);
#5601=ORIENTED_EDGE('',*,*,#4453,.F.);
#5602=ORIENTED_EDGE('',*,*,#4454,.T.);
#5603=ORIENTED_EDGE('',*,*,#4455,.F.);
#5604=ORIENTED_EDGE('',*,*,#4451,.F.);
#5605=ORIENTED_EDGE('',*,*,#4456,.F.);
#5606=ORIENTED_EDGE('',*,*,#4457,.T.);
#5607=ORIENTED_EDGE('',*,*,#4458,.F.);
#5608=ORIENTED_EDGE('',*,*,#4454,.F.);
#5609=ORIENTED_EDGE('',*,*,#4459,.F.);
#5610=ORIENTED_EDGE('',*,*,#4460,.T.);
#5611=ORIENTED_EDGE('',*,*,#4461,.F.);
#5612=ORIENTED_EDGE('',*,*,#4457,.F.);
#5613=ORIENTED_EDGE('',*,*,#4407,.T.);
#5614=ORIENTED_EDGE('',*,*,#4462,.F.);
#5615=ORIENTED_EDGE('',*,*,#4463,.T.);
#5616=ORIENTED_EDGE('',*,*,#4464,.F.);
#5617=ORIENTED_EDGE('',*,*,#4460,.F.);
#5618=ORIENTED_EDGE('',*,*,#4465,.F.);
#5619=ORIENTED_EDGE('',*,*,#4466,.T.);
#5620=ORIENTED_EDGE('',*,*,#4467,.F.);
#5621=ORIENTED_EDGE('',*,*,#4463,.F.);
#5622=ORIENTED_EDGE('',*,*,#4468,.F.);
#5623=ORIENTED_EDGE('',*,*,#4469,.T.);
#5624=ORIENTED_EDGE('',*,*,#4470,.F.);
#5625=ORIENTED_EDGE('',*,*,#4466,.F.);
#5626=ORIENTED_EDGE('',*,*,#4471,.F.);
#5627=ORIENTED_EDGE('',*,*,#4472,.F.);
#5628=ORIENTED_EDGE('',*,*,#4473,.F.);
#5629=ORIENTED_EDGE('',*,*,#4469,.F.);
#5630=ORIENTED_EDGE('',*,*,#4474,.F.);
#5631=ORIENTED_EDGE('',*,*,#4475,.T.);
#5632=ORIENTED_EDGE('',*,*,#4476,.F.);
#5633=ORIENTED_EDGE('',*,*,#4477,.F.);
#5634=ORIENTED_EDGE('',*,*,#4478,.F.);
#5635=ORIENTED_EDGE('',*,*,#4479,.T.);
#5636=ORIENTED_EDGE('',*,*,#4480,.F.);
#5637=ORIENTED_EDGE('',*,*,#4475,.F.);
#5638=ORIENTED_EDGE('',*,*,#4481,.F.);
#5639=ORIENTED_EDGE('',*,*,#4482,.T.);
#5640=ORIENTED_EDGE('',*,*,#4483,.F.);
#5641=ORIENTED_EDGE('',*,*,#4479,.F.);
#5642=ORIENTED_EDGE('',*,*,#4484,.F.);
#5643=ORIENTED_EDGE('',*,*,#4485,.T.);
#5644=ORIENTED_EDGE('',*,*,#4486,.F.);
#5645=ORIENTED_EDGE('',*,*,#4482,.F.);
#5646=ORIENTED_EDGE('',*,*,#4487,.F.);
#5647=ORIENTED_EDGE('',*,*,#4488,.T.);
#5648=ORIENTED_EDGE('',*,*,#4489,.F.);
#5649=ORIENTED_EDGE('',*,*,#4485,.F.);
#5650=ORIENTED_EDGE('',*,*,#4490,.F.);
#5651=ORIENTED_EDGE('',*,*,#4491,.T.);
#5652=ORIENTED_EDGE('',*,*,#4492,.F.);
#5653=ORIENTED_EDGE('',*,*,#4488,.F.);
#5654=ORIENTED_EDGE('',*,*,#4493,.F.);
#5655=ORIENTED_EDGE('',*,*,#4494,.T.);
#5656=ORIENTED_EDGE('',*,*,#4495,.F.);
#5657=ORIENTED_EDGE('',*,*,#4491,.F.);
#5658=ORIENTED_EDGE('',*,*,#4496,.F.);
#5659=ORIENTED_EDGE('',*,*,#4497,.T.);
#5660=ORIENTED_EDGE('',*,*,#4498,.F.);
#5661=ORIENTED_EDGE('',*,*,#4494,.F.);
#5662=ORIENTED_EDGE('',*,*,#4499,.F.);
#5663=ORIENTED_EDGE('',*,*,#4500,.F.);
#5664=ORIENTED_EDGE('',*,*,#4501,.F.);
#5665=ORIENTED_EDGE('',*,*,#4497,.F.);
#5666=ORIENTED_EDGE('',*,*,#4502,.F.);
#5667=ORIENTED_EDGE('',*,*,#4503,.T.);
#5668=ORIENTED_EDGE('',*,*,#4504,.F.);
#5669=ORIENTED_EDGE('',*,*,#4505,.F.);
#5670=ORIENTED_EDGE('',*,*,#4506,.F.);
#5671=ORIENTED_EDGE('',*,*,#4507,.T.);
#5672=ORIENTED_EDGE('',*,*,#4508,.F.);
#5673=ORIENTED_EDGE('',*,*,#4503,.F.);
#5674=ORIENTED_EDGE('',*,*,#4509,.F.);
#5675=ORIENTED_EDGE('',*,*,#4510,.T.);
#5676=ORIENTED_EDGE('',*,*,#4511,.F.);
#5677=ORIENTED_EDGE('',*,*,#4507,.F.);
#5678=ORIENTED_EDGE('',*,*,#4512,.F.);
#5679=ORIENTED_EDGE('',*,*,#4513,.T.);
#5680=ORIENTED_EDGE('',*,*,#4514,.F.);
#5681=ORIENTED_EDGE('',*,*,#4510,.F.);
#5682=ORIENTED_EDGE('',*,*,#4515,.F.);
#5683=ORIENTED_EDGE('',*,*,#4516,.T.);
#5684=ORIENTED_EDGE('',*,*,#4517,.F.);
#5685=ORIENTED_EDGE('',*,*,#4513,.F.);
#5686=ORIENTED_EDGE('',*,*,#4411,.T.);
#5687=ORIENTED_EDGE('',*,*,#4518,.F.);
#5688=ORIENTED_EDGE('',*,*,#4519,.T.);
#5689=ORIENTED_EDGE('',*,*,#4520,.F.);
#5690=ORIENTED_EDGE('',*,*,#4516,.F.);
#5691=ORIENTED_EDGE('',*,*,#4521,.F.);
#5692=ORIENTED_EDGE('',*,*,#4522,.T.);
#5693=ORIENTED_EDGE('',*,*,#4523,.F.);
#5694=ORIENTED_EDGE('',*,*,#4519,.F.);
#5695=ORIENTED_EDGE('',*,*,#4524,.F.);
#5696=ORIENTED_EDGE('',*,*,#4525,.T.);
#5697=ORIENTED_EDGE('',*,*,#4526,.F.);
#5698=ORIENTED_EDGE('',*,*,#4522,.F.);
#5699=ORIENTED_EDGE('',*,*,#4527,.F.);
#5700=ORIENTED_EDGE('',*,*,#4528,.F.);
#5701=ORIENTED_EDGE('',*,*,#4529,.F.);
#5702=ORIENTED_EDGE('',*,*,#4525,.F.);
#5703=ORIENTED_EDGE('',*,*,#4414,.T.);
#5704=ORIENTED_EDGE('',*,*,#4530,.T.);
#5705=ORIENTED_EDGE('',*,*,#4531,.F.);
#5706=ORIENTED_EDGE('',*,*,#4530,.F.);
#5707=ORIENTED_EDGE('',*,*,#4415,.T.);
#5708=ORIENTED_EDGE('',*,*,#4444,.T.);
#5709=ORIENTED_EDGE('',*,*,#4532,.T.);
#5710=ORIENTED_EDGE('',*,*,#4533,.T.);
#5711=ORIENTED_EDGE('',*,*,#4534,.F.);
#5712=ORIENTED_EDGE('',*,*,#4421,.T.);
#5713=ORIENTED_EDGE('',*,*,#4535,.F.);
#5714=ORIENTED_EDGE('',*,*,#4536,.F.);
#5715=ORIENTED_EDGE('',*,*,#4537,.T.);
#5716=ORIENTED_EDGE('',*,*,#4472,.T.);
#5717=ORIENTED_EDGE('',*,*,#4538,.T.);
#5718=ORIENTED_EDGE('',*,*,#4536,.T.);
#5719=ORIENTED_EDGE('',*,*,#4539,.F.);
#5720=ORIENTED_EDGE('',*,*,#4449,.T.);
#5721=ORIENTED_EDGE('',*,*,#4540,.F.);
#5722=ORIENTED_EDGE('',*,*,#4541,.F.);
#5723=ORIENTED_EDGE('',*,*,#4542,.T.);
#5724=ORIENTED_EDGE('',*,*,#4500,.T.);
#5725=ORIENTED_EDGE('',*,*,#4543,.T.);
#5726=ORIENTED_EDGE('',*,*,#4541,.T.);
#5727=ORIENTED_EDGE('',*,*,#4544,.F.);
#5728=ORIENTED_EDGE('',*,*,#4477,.T.);
#5729=ORIENTED_EDGE('',*,*,#4545,.F.);
#5730=ORIENTED_EDGE('',*,*,#4546,.F.);
#5731=ORIENTED_EDGE('',*,*,#4547,.T.);
#5732=ORIENTED_EDGE('',*,*,#4528,.T.);
#5733=ORIENTED_EDGE('',*,*,#4548,.T.);
#5734=ORIENTED_EDGE('',*,*,#4546,.T.);
#5735=ORIENTED_EDGE('',*,*,#4549,.F.);
#5736=ORIENTED_EDGE('',*,*,#4505,.T.);
#5737=ORIENTED_EDGE('',*,*,#4550,.F.);
#5738=ORIENTED_EDGE('',*,*,#4533,.F.);
#5739=ORIENTED_EDGE('',*,*,#4551,.T.);
#5740=ORIENTED_EDGE('',*,*,#4420,.T.);
#5741=ORIENTED_EDGE('',*,*,#4424,.T.);
#5742=ORIENTED_EDGE('',*,*,#4427,.T.);
#5743=ORIENTED_EDGE('',*,*,#4430,.T.);
#5744=ORIENTED_EDGE('',*,*,#4433,.T.);
#5745=ORIENTED_EDGE('',*,*,#4436,.T.);
#5746=ORIENTED_EDGE('',*,*,#4439,.T.);
#5747=ORIENTED_EDGE('',*,*,#4442,.T.);
#5748=ORIENTED_EDGE('',*,*,#4445,.T.);
#5749=ORIENTED_EDGE('',*,*,#4534,.T.);
#5750=ORIENTED_EDGE('',*,*,#4550,.T.);
#5751=ORIENTED_EDGE('',*,*,#4504,.T.);
#5752=ORIENTED_EDGE('',*,*,#4508,.T.);
#5753=ORIENTED_EDGE('',*,*,#4511,.T.);
#5754=ORIENTED_EDGE('',*,*,#4514,.T.);
#5755=ORIENTED_EDGE('',*,*,#4517,.T.);
#5756=ORIENTED_EDGE('',*,*,#4520,.T.);
#5757=ORIENTED_EDGE('',*,*,#4523,.T.);
#5758=ORIENTED_EDGE('',*,*,#4526,.T.);
#5759=ORIENTED_EDGE('',*,*,#4529,.T.);
#5760=ORIENTED_EDGE('',*,*,#4549,.T.);
#5761=ORIENTED_EDGE('',*,*,#4545,.T.);
#5762=ORIENTED_EDGE('',*,*,#4476,.T.);
#5763=ORIENTED_EDGE('',*,*,#4480,.T.);
#5764=ORIENTED_EDGE('',*,*,#4483,.T.);
#5765=ORIENTED_EDGE('',*,*,#4486,.T.);
#5766=ORIENTED_EDGE('',*,*,#4489,.T.);
#5767=ORIENTED_EDGE('',*,*,#4492,.T.);
#5768=ORIENTED_EDGE('',*,*,#4495,.T.);
#5769=ORIENTED_EDGE('',*,*,#4498,.T.);
#5770=ORIENTED_EDGE('',*,*,#4501,.T.);
#5771=ORIENTED_EDGE('',*,*,#4544,.T.);
#5772=ORIENTED_EDGE('',*,*,#4540,.T.);
#5773=ORIENTED_EDGE('',*,*,#4448,.T.);
#5774=ORIENTED_EDGE('',*,*,#4452,.T.);
#5775=ORIENTED_EDGE('',*,*,#4455,.T.);
#5776=ORIENTED_EDGE('',*,*,#4458,.T.);
#5777=ORIENTED_EDGE('',*,*,#4461,.T.);
#5778=ORIENTED_EDGE('',*,*,#4464,.T.);
#5779=ORIENTED_EDGE('',*,*,#4467,.T.);
#5780=ORIENTED_EDGE('',*,*,#4470,.T.);
#5781=ORIENTED_EDGE('',*,*,#4473,.T.);
#5782=ORIENTED_EDGE('',*,*,#4539,.T.);
#5783=ORIENTED_EDGE('',*,*,#4535,.T.);
#5784=ORIENTED_EDGE('',*,*,#4531,.T.);
#5785=ORIENTED_EDGE('',*,*,#4418,.T.);
#5786=ORIENTED_EDGE('',*,*,#4537,.F.);
#5787=ORIENTED_EDGE('',*,*,#4538,.F.);
#5788=ORIENTED_EDGE('',*,*,#4471,.T.);
#5789=ORIENTED_EDGE('',*,*,#4468,.T.);
#5790=ORIENTED_EDGE('',*,*,#4465,.T.);
#5791=ORIENTED_EDGE('',*,*,#4462,.T.);
#5792=ORIENTED_EDGE('',*,*,#4459,.T.);
#5793=ORIENTED_EDGE('',*,*,#4456,.T.);
#5794=ORIENTED_EDGE('',*,*,#4453,.T.);
#5795=ORIENTED_EDGE('',*,*,#4450,.T.);
#5796=ORIENTED_EDGE('',*,*,#4446,.T.);
#5797=ORIENTED_EDGE('',*,*,#4542,.F.);
#5798=ORIENTED_EDGE('',*,*,#4543,.F.);
#5799=ORIENTED_EDGE('',*,*,#4499,.T.);
#5800=ORIENTED_EDGE('',*,*,#4496,.T.);
#5801=ORIENTED_EDGE('',*,*,#4493,.T.);
#5802=ORIENTED_EDGE('',*,*,#4490,.T.);
#5803=ORIENTED_EDGE('',*,*,#4487,.T.);
#5804=ORIENTED_EDGE('',*,*,#4484,.T.);
#5805=ORIENTED_EDGE('',*,*,#4481,.T.);
#5806=ORIENTED_EDGE('',*,*,#4478,.T.);
#5807=ORIENTED_EDGE('',*,*,#4474,.T.);
#5808=ORIENTED_EDGE('',*,*,#4547,.F.);
#5809=ORIENTED_EDGE('',*,*,#4548,.F.);
#5810=ORIENTED_EDGE('',*,*,#4527,.T.);
#5811=ORIENTED_EDGE('',*,*,#4524,.T.);
#5812=ORIENTED_EDGE('',*,*,#4521,.T.);
#5813=ORIENTED_EDGE('',*,*,#4518,.T.);
#5814=ORIENTED_EDGE('',*,*,#4515,.T.);
#5815=ORIENTED_EDGE('',*,*,#4512,.T.);
#5816=ORIENTED_EDGE('',*,*,#4509,.T.);
#5817=ORIENTED_EDGE('',*,*,#4506,.T.);
#5818=ORIENTED_EDGE('',*,*,#4502,.T.);
#5819=ORIENTED_EDGE('',*,*,#4551,.F.);
#5820=ORIENTED_EDGE('',*,*,#4532,.F.);
#5821=ORIENTED_EDGE('',*,*,#4443,.T.);
#5822=ORIENTED_EDGE('',*,*,#4440,.T.);
#5823=ORIENTED_EDGE('',*,*,#4437,.T.);
#5824=ORIENTED_EDGE('',*,*,#4434,.T.);
#5825=ORIENTED_EDGE('',*,*,#4431,.T.);
#5826=ORIENTED_EDGE('',*,*,#4428,.T.);
#5827=ORIENTED_EDGE('',*,*,#4425,.T.);
#5828=ORIENTED_EDGE('',*,*,#4422,.T.);
#5829=ORIENTED_EDGE('',*,*,#4416,.T.);
#7137=CYLINDRICAL_SURFACE('',#8124,0.275);
#7138=CYLINDRICAL_SURFACE('',#8127,0.21);
#7139=CYLINDRICAL_SURFACE('',#8165,0.21);
#7267=ADVANCED_FACE('',(#1066,#622),#7137,.F.);
#7268=ADVANCED_FACE('',(#1067),#7138,.F.);
#7269=ADVANCED_FACE('',(#1068),#754,.F.);
#7270=ADVANCED_FACE('',(#1069),#755,.F.);
#7271=ADVANCED_FACE('',(#1070),#756,.F.);
#7272=ADVANCED_FACE('',(#1071),#757,.F.);
#7273=ADVANCED_FACE('',(#1072),#758,.F.);
#7274=ADVANCED_FACE('',(#1073),#759,.F.);
#7275=ADVANCED_FACE('',(#1074),#760,.F.);
#7276=ADVANCED_FACE('',(#1075),#761,.F.);
#7277=ADVANCED_FACE('',(#1076),#762,.F.);
#7278=ADVANCED_FACE('',(#1077),#763,.F.);
#7279=ADVANCED_FACE('',(#1078),#764,.F.);
#7280=ADVANCED_FACE('',(#1079),#765,.F.);
#7281=ADVANCED_FACE('',(#1080),#766,.F.);
#7282=ADVANCED_FACE('',(#1081,#623),#767,.F.);
#7283=ADVANCED_FACE('',(#1082),#768,.F.);
#7284=ADVANCED_FACE('',(#1083),#769,.F.);
#7285=ADVANCED_FACE('',(#1084),#770,.F.);
#7286=ADVANCED_FACE('',(#1085),#771,.F.);
#7287=ADVANCED_FACE('',(#1086),#772,.F.);
#7288=ADVANCED_FACE('',(#1087),#773,.F.);
#7289=ADVANCED_FACE('',(#1088),#774,.F.);
#7290=ADVANCED_FACE('',(#1089),#775,.F.);
#7291=ADVANCED_FACE('',(#1090),#776,.F.);
#7292=ADVANCED_FACE('',(#1091),#777,.F.);
#7293=ADVANCED_FACE('',(#1092),#778,.F.);
#7294=ADVANCED_FACE('',(#1093),#779,.F.);
#7295=ADVANCED_FACE('',(#1094),#780,.F.);
#7296=ADVANCED_FACE('',(#1095),#781,.F.);
#7297=ADVANCED_FACE('',(#1096),#782,.F.);
#7298=ADVANCED_FACE('',(#1097),#783,.F.);
#7299=ADVANCED_FACE('',(#1098),#784,.F.);
#7300=ADVANCED_FACE('',(#1099,#624),#785,.F.);
#7301=ADVANCED_FACE('',(#1100),#786,.F.);
#7302=ADVANCED_FACE('',(#1101),#787,.F.);
#7303=ADVANCED_FACE('',(#1102),#788,.F.);
#7304=ADVANCED_FACE('',(#1103),#789,.F.);
#7305=ADVANCED_FACE('',(#1104),#7139,.F.);
#7306=ADVANCED_FACE('',(#1105),#790,.T.);
#7307=ADVANCED_FACE('',(#1106),#791,.T.);
#7308=ADVANCED_FACE('',(#1107),#792,.T.);
#7309=ADVANCED_FACE('',(#1108),#793,.T.);
#7310=ADVANCED_FACE('',(#1109),#794,.T.);
#7311=ADVANCED_FACE('',(#1110),#795,.T.);
#7312=ADVANCED_FACE('',(#1111),#796,.T.);
#7313=ADVANCED_FACE('',(#1112),#797,.T.);
#7314=ADVANCED_FACE('',(#1113,#625),#798,.T.);
#7315=ADVANCED_FACE('',(#1114,#626),#799,.F.);
#7629=CLOSED_SHELL('',(#7267,#7268,#7269,#7270,#7271,#7272,#7273,#7274,
#7275,#7276,#7277,#7278,#7279,#7280,#7281,#7282,#7283,#7284,#7285,#7286,
#7287,#7288,#7289,#7290,#7291,#7292,#7293,#7294,#7295,#7296,#7297,#7298,
#7299,#7300,#7301,#7302,#7303,#7304,#7305,#7306,#7307,#7308,#7309,#7310,
#7311,#7312,#7313,#7314,#7315));
#8123=AXIS2_PLACEMENT_3D('',#11503,#9119,#9120);
#8124=AXIS2_PLACEMENT_3D('',#11504,#9121,#9122);
#8125=AXIS2_PLACEMENT_3D('',#11506,#9123,#9124);
#8126=AXIS2_PLACEMENT_3D('',#11534,#9127,#9128);
#8127=AXIS2_PLACEMENT_3D('',#11606,#9129,#9130);
#8128=AXIS2_PLACEMENT_3D('',#11608,#9131,#9132);
#8129=AXIS2_PLACEMENT_3D('',#11610,#9134,#9135);
#8130=AXIS2_PLACEMENT_3D('',#11619,#9140,#9141);
#8131=AXIS2_PLACEMENT_3D('',#11625,#9145,#9146);
#8132=AXIS2_PLACEMENT_3D('',#11631,#9150,#9151);
#8133=AXIS2_PLACEMENT_3D('',#11637,#9155,#9156);
#8134=AXIS2_PLACEMENT_3D('',#11643,#9160,#9161);
#8135=AXIS2_PLACEMENT_3D('',#11649,#9165,#9166);
#8136=AXIS2_PLACEMENT_3D('',#11655,#9170,#9171);
#8137=AXIS2_PLACEMENT_3D('',#11661,#9175,#9176);
#8138=AXIS2_PLACEMENT_3D('',#11667,#9180,#9181);
#8139=AXIS2_PLACEMENT_3D('',#11676,#9186,#9187);
#8140=AXIS2_PLACEMENT_3D('',#11682,#9191,#9192);
#8141=AXIS2_PLACEMENT_3D('',#11688,#9196,#9197);
#8142=AXIS2_PLACEMENT_3D('',#11694,#9201,#9202);
#8143=AXIS2_PLACEMENT_3D('',#11700,#9206,#9207);
#8144=AXIS2_PLACEMENT_3D('',#11706,#9211,#9212);
#8145=AXIS2_PLACEMENT_3D('',#11712,#9216,#9217);
#8146=AXIS2_PLACEMENT_3D('',#11718,#9221,#9222);
#8147=AXIS2_PLACEMENT_3D('',#11724,#9226,#9227);
#8148=AXIS2_PLACEMENT_3D('',#11733,#9232,#9233);
#8149=AXIS2_PLACEMENT_3D('',#11739,#9237,#9238);
#8150=AXIS2_PLACEMENT_3D('',#11745,#9242,#9243);
#8151=AXIS2_PLACEMENT_3D('',#11751,#9247,#9248);
#8152=AXIS2_PLACEMENT_3D('',#11757,#9252,#9253);
#8153=AXIS2_PLACEMENT_3D('',#11763,#9257,#9258);
#8154=AXIS2_PLACEMENT_3D('',#11769,#9262,#9263);
#8155=AXIS2_PLACEMENT_3D('',#11775,#9267,#9268);
#8156=AXIS2_PLACEMENT_3D('',#11781,#9272,#9273);
#8157=AXIS2_PLACEMENT_3D('',#11790,#9278,#9279);
#8158=AXIS2_PLACEMENT_3D('',#11796,#9283,#9284);
#8159=AXIS2_PLACEMENT_3D('',#11802,#9288,#9289);
#8160=AXIS2_PLACEMENT_3D('',#11808,#9293,#9294);
#8161=AXIS2_PLACEMENT_3D('',#11814,#9298,#9299);
#8162=AXIS2_PLACEMENT_3D('',#11820,#9303,#9304);
#8163=AXIS2_PLACEMENT_3D('',#11826,#9308,#9309);
#8164=AXIS2_PLACEMENT_3D('',#11832,#9313,#9314);
#8165=AXIS2_PLACEMENT_3D('',#11838,#9318,#9319);
#8166=AXIS2_PLACEMENT_3D('',#11841,#9321,#9322);
#8167=AXIS2_PLACEMENT_3D('',#11842,#9323,#9324);
#8168=AXIS2_PLACEMENT_3D('',#11848,#9328,#9329);
#8169=AXIS2_PLACEMENT_3D('',#11854,#9333,#9334);
#8170=AXIS2_PLACEMENT_3D('',#11857,#9337,#9338);
#8171=AXIS2_PLACEMENT_3D('',#11863,#9342,#9343);
#8172=AXIS2_PLACEMENT_3D('',#11866,#9346,#9347);
#8173=AXIS2_PLACEMENT_3D('',#11872,#9351,#9352);
#8174=AXIS2_PLACEMENT_3D('',#11875,#9355,#9356);
#8175=AXIS2_PLACEMENT_3D('',#11878,#9359,#9360);
#8176=AXIS2_PLACEMENT_3D('',#11879,#9361,#9362);
#9119=DIRECTION('axis',(0.,0.,1.));
#9120=DIRECTION('refdir',(1.,0.,0.));
#9121=DIRECTION('center_axis',(0.,0.,1.));
#9122=DIRECTION('ref_axis',(1.,0.,0.));
#9123=DIRECTION('center_axis',(0.,0.,1.));
#9124=DIRECTION('ref_axis',(1.,0.,0.));
#9125=DIRECTION('',(0.,0.,1.));
#9126=DIRECTION('',(0.,0.,1.));
#9127=DIRECTION('center_axis',(0.,0.,-1.));
#9128=DIRECTION('ref_axis',(1.,0.,0.));
#9129=DIRECTION('center_axis',(1.,0.,0.));
#9130=DIRECTION('ref_axis',(0.,0.,-1.));
#9131=DIRECTION('center_axis',(1.,0.,0.));
#9132=DIRECTION('ref_axis',(0.,0.,-1.));
#9133=DIRECTION('',(1.,0.,0.));
#9134=DIRECTION('center_axis',(0.,0.,-1.));
#9135=DIRECTION('ref_axis',(0.,1.,0.));
#9136=DIRECTION('',(0.,1.,0.));
#9137=DIRECTION('',(1.,0.,0.));
#9138=DIRECTION('',(0.,-1.,0.));
#9139=DIRECTION('',(1.,0.,0.));
#9140=DIRECTION('center_axis',(0.,1.,-8.88178419700125E-16));
#9141=DIRECTION('ref_axis',(0.,8.88178419700125E-16,1.));
#9142=DIRECTION('',(0.,8.88178419700125E-16,1.));
#9143=DIRECTION('',(1.,0.,0.));
#9144=DIRECTION('',(0.,-8.88178419700125E-16,-1.));
#9145=DIRECTION('center_axis',(0.,-7.40148683083439E-16,-1.));
#9146=DIRECTION('ref_axis',(0.,1.,-7.40148683083439E-16));
#9147=DIRECTION('',(0.,1.,-7.40148683083439E-16));
#9148=DIRECTION('',(1.,0.,0.));
#9149=DIRECTION('',(0.,-1.,7.40148683083439E-16));
#9150=DIRECTION('center_axis',(0.,-0.707106781186547,-0.707106781186548));
#9151=DIRECTION('ref_axis',(0.,0.707106781186548,-0.707106781186547));
#9152=DIRECTION('',(0.,0.707106781186548,-0.707106781186547));
#9153=DIRECTION('',(1.,0.,0.));
#9154=DIRECTION('',(0.,-0.707106781186548,0.707106781186547));
#9155=DIRECTION('center_axis',(0.,-1.,2.77555756156289E-16));
#9156=DIRECTION('ref_axis',(0.,-2.77555756156289E-16,-1.));
#9157=DIRECTION('',(0.,-2.77555756156289E-16,-1.));
#9158=DIRECTION('',(1.,0.,0.));
#9159=DIRECTION('',(0.,2.77555756156289E-16,1.));
#9160=DIRECTION('center_axis',(0.,-0.707106781186547,0.707106781186548));
#9161=DIRECTION('ref_axis',(0.,-0.707106781186548,-0.707106781186547));
#9162=DIRECTION('',(0.,-0.707106781186548,-0.707106781186547));
#9163=DIRECTION('',(1.,0.,0.));
#9164=DIRECTION('',(0.,0.707106781186548,0.707106781186547));
#9165=DIRECTION('center_axis',(0.,7.40148683083438E-16,1.));
#9166=DIRECTION('ref_axis',(0.,-1.,7.40148683083438E-16));
#9167=DIRECTION('',(0.,-1.,7.40148683083438E-16));
#9168=DIRECTION('',(1.,0.,0.));
#9169=DIRECTION('',(0.,1.,-7.40148683083438E-16));
#9170=DIRECTION('center_axis',(0.,1.,-4.44089209850063E-16));
#9171=DIRECTION('ref_axis',(0.,4.44089209850063E-16,1.));
#9172=DIRECTION('',(0.,4.44089209850063E-16,1.));
#9173=DIRECTION('',(1.,0.,0.));
#9174=DIRECTION('',(0.,-4.44089209850063E-16,-1.));
#9175=DIRECTION('center_axis',(0.,2.41352831440251E-16,1.));
#9176=DIRECTION('ref_axis',(0.,-1.,2.41352831440251E-16));
#9177=DIRECTION('',(0.,-1.,2.41352831440251E-16));
#9178=DIRECTION('',(-1.,0.,0.));
#9179=DIRECTION('',(0.,1.,-2.41352831440251E-16));
#9180=DIRECTION('center_axis',(0.,-1.,2.41352831440251E-16));
#9181=DIRECTION('ref_axis',(0.,-2.41352831440251E-16,-1.));
#9182=DIRECTION('',(0.,-2.41352831440251E-16,-1.));
#9183=DIRECTION('',(1.,0.,0.));
#9184=DIRECTION('',(0.,2.41352831440251E-16,1.));
#9185=DIRECTION('',(1.,0.,0.));
#9186=DIRECTION('center_axis',(0.,0.,-1.));
#9187=DIRECTION('ref_axis',(0.,1.,0.));
#9188=DIRECTION('',(0.,1.,0.));
#9189=DIRECTION('',(1.,0.,0.));
#9190=DIRECTION('',(0.,-1.,0.));
#9191=DIRECTION('center_axis',(0.,-1.,0.));
#9192=DIRECTION('ref_axis',(0.,0.,-1.));
#9193=DIRECTION('',(0.,0.,-1.));
#9194=DIRECTION('',(1.,0.,0.));
#9195=DIRECTION('',(0.,0.,1.));
#9196=DIRECTION('center_axis',(0.,-0.707106781186547,0.707106781186548));
#9197=DIRECTION('ref_axis',(0.,-0.707106781186548,-0.707106781186547));
#9198=DIRECTION('',(0.,-0.707106781186548,-0.707106781186547));
#9199=DIRECTION('',(1.,0.,0.));
#9200=DIRECTION('',(0.,0.707106781186548,0.707106781186547));
#9201=DIRECTION('center_axis',(0.,0.,1.));
#9202=DIRECTION('ref_axis',(0.,-1.,0.));
#9203=DIRECTION('',(0.,-1.,0.));
#9204=DIRECTION('',(1.,0.,0.));
#9205=DIRECTION('',(0.,1.,0.));
#9206=DIRECTION('center_axis',(0.,0.707106781186548,0.707106781186547));
#9207=DIRECTION('ref_axis',(0.,-0.707106781186547,0.707106781186548));
#9208=DIRECTION('',(0.,-0.707106781186547,0.707106781186548));
#9209=DIRECTION('',(1.,0.,0.));
#9210=DIRECTION('',(0.,0.707106781186547,-0.707106781186548));
#9211=DIRECTION('center_axis',(0.,1.,0.));
#9212=DIRECTION('ref_axis',(0.,0.,1.));
#9213=DIRECTION('',(0.,0.,1.));
#9214=DIRECTION('',(1.,0.,0.));
#9215=DIRECTION('',(0.,0.,-1.));
#9216=DIRECTION('center_axis',(0.,0.,-1.));
#9217=DIRECTION('ref_axis',(0.,1.,0.));
#9218=DIRECTION('',(0.,1.,0.));
#9219=DIRECTION('',(1.,0.,0.));
#9220=DIRECTION('',(0.,-1.,0.));
#9221=DIRECTION('center_axis',(0.,1.,-2.41352831440251E-16));
#9222=DIRECTION('ref_axis',(0.,2.41352831440251E-16,1.));
#9223=DIRECTION('',(0.,2.41352831440251E-16,1.));
#9224=DIRECTION('',(-1.,0.,0.));
#9225=DIRECTION('',(0.,-2.41352831440251E-16,-1.));
#9226=DIRECTION('center_axis',(0.,0.,1.));
#9227=DIRECTION('ref_axis',(0.,-1.,0.));
#9228=DIRECTION('',(0.,-1.,0.));
#9229=DIRECTION('',(1.,0.,0.));
#9230=DIRECTION('',(0.,1.,0.));
#9231=DIRECTION('',(1.,0.,0.));
#9232=DIRECTION('center_axis',(0.,-1.,0.));
#9233=DIRECTION('ref_axis',(0.,0.,-1.));
#9234=DIRECTION('',(0.,0.,-1.));
#9235=DIRECTION('',(1.,0.,0.));
#9236=DIRECTION('',(0.,0.,1.));
#9237=DIRECTION('center_axis',(0.,0.,1.));
#9238=DIRECTION('ref_axis',(0.,-1.,0.));
#9239=DIRECTION('',(0.,-1.,0.));
#9240=DIRECTION('',(1.,0.,0.));
#9241=DIRECTION('',(0.,1.,0.));
#9242=DIRECTION('center_axis',(0.,0.707106781186548,0.707106781186548));
#9243=DIRECTION('ref_axis',(0.,-0.707106781186548,0.707106781186548));
#9244=DIRECTION('',(0.,-0.707106781186548,0.707106781186548));
#9245=DIRECTION('',(1.,0.,0.));
#9246=DIRECTION('',(0.,0.707106781186548,-0.707106781186548));
#9247=DIRECTION('center_axis',(0.,1.,0.));
#9248=DIRECTION('ref_axis',(0.,0.,1.));
#9249=DIRECTION('',(0.,0.,1.));
#9250=DIRECTION('',(1.,0.,0.));
#9251=DIRECTION('',(0.,0.,-1.));
#9252=DIRECTION('center_axis',(0.,0.707106781186548,-0.707106781186547));
#9253=DIRECTION('ref_axis',(0.,0.707106781186547,0.707106781186548));
#9254=DIRECTION('',(0.,0.707106781186547,0.707106781186548));
#9255=DIRECTION('',(1.,0.,0.));
#9256=DIRECTION('',(0.,-0.707106781186547,-0.707106781186548));
#9257=DIRECTION('center_axis',(0.,-7.40148683083438E-16,-1.));
#9258=DIRECTION('ref_axis',(0.,1.,-7.40148683083438E-16));
#9259=DIRECTION('',(0.,1.,-7.40148683083438E-16));
#9260=DIRECTION('',(1.,0.,0.));
#9261=DIRECTION('',(0.,-1.,7.40148683083438E-16));
#9262=DIRECTION('center_axis',(0.,-1.,0.));
#9263=DIRECTION('ref_axis',(0.,0.,-1.));
#9264=DIRECTION('',(0.,0.,-1.));
#9265=DIRECTION('',(1.,0.,0.));
#9266=DIRECTION('',(0.,0.,1.));
#9267=DIRECTION('center_axis',(0.,0.,-1.));
#9268=DIRECTION('ref_axis',(0.,1.,0.));
#9269=DIRECTION('',(0.,1.,0.));
#9270=DIRECTION('',(-1.,0.,0.));
#9271=DIRECTION('',(0.,-1.,0.));
#9272=DIRECTION('center_axis',(0.,1.,0.));
#9273=DIRECTION('ref_axis',(0.,0.,1.));
#9274=DIRECTION('',(0.,0.,1.));
#9275=DIRECTION('',(1.,0.,0.));
#9276=DIRECTION('',(0.,0.,-1.));
#9277=DIRECTION('',(1.,0.,0.));
#9278=DIRECTION('center_axis',(0.,0.,1.));
#9279=DIRECTION('ref_axis',(0.,-1.,0.));
#9280=DIRECTION('',(0.,-1.,0.));
#9281=DIRECTION('',(1.,0.,0.));
#9282=DIRECTION('',(0.,1.,0.));
#9283=DIRECTION('center_axis',(0.,1.,0.));
#9284=DIRECTION('ref_axis',(0.,0.,1.));
#9285=DIRECTION('',(0.,0.,1.));
#9286=DIRECTION('',(1.,0.,0.));
#9287=DIRECTION('',(0.,0.,-1.));
#9288=DIRECTION('center_axis',(0.,0.707106781186547,-0.707106781186548));
#9289=DIRECTION('ref_axis',(0.,0.707106781186548,0.707106781186547));
#9290=DIRECTION('',(0.,0.707106781186548,0.707106781186547));
#9291=DIRECTION('',(1.,0.,0.));
#9292=DIRECTION('',(0.,-0.707106781186548,-0.707106781186547));
#9293=DIRECTION('center_axis',(0.,0.,-1.));
#9294=DIRECTION('ref_axis',(0.,1.,0.));
#9295=DIRECTION('',(0.,1.,0.));
#9296=DIRECTION('',(1.,0.,0.));
#9297=DIRECTION('',(0.,-1.,0.));
#9298=DIRECTION('center_axis',(0.,-0.707106781186547,-0.707106781186548));
#9299=DIRECTION('ref_axis',(0.,0.707106781186548,-0.707106781186547));
#9300=DIRECTION('',(0.,0.707106781186548,-0.707106781186547));
#9301=DIRECTION('',(1.,0.,0.));
#9302=DIRECTION('',(0.,-0.707106781186548,0.707106781186547));
#9303=DIRECTION('center_axis',(0.,-1.,0.));
#9304=DIRECTION('ref_axis',(0.,0.,-1.));
#9305=DIRECTION('',(0.,0.,-1.));
#9306=DIRECTION('',(1.,0.,0.));
#9307=DIRECTION('',(0.,0.,1.));
#9308=DIRECTION('center_axis',(0.,0.,1.));
#9309=DIRECTION('ref_axis',(0.,-1.,0.));
#9310=DIRECTION('',(0.,-1.,0.));
#9311=DIRECTION('',(1.,0.,0.));
#9312=DIRECTION('',(0.,1.,0.));
#9313=DIRECTION('center_axis',(0.,-1.,0.));
#9314=DIRECTION('ref_axis',(0.,0.,-1.));
#9315=DIRECTION('',(0.,0.,-1.));
#9316=DIRECTION('',(-1.,0.,0.));
#9317=DIRECTION('',(0.,0.,1.));
#9318=DIRECTION('center_axis',(1.,0.,0.));
#9319=DIRECTION('ref_axis',(0.,0.,-1.));
#9320=DIRECTION('',(1.,0.,0.));
#9321=DIRECTION('center_axis',(-1.,0.,0.));
#9322=DIRECTION('ref_axis',(0.,0.,-1.));
#9323=DIRECTION('center_axis',(0.,1.,0.));
#9324=DIRECTION('ref_axis',(0.,0.,1.));
#9325=DIRECTION('',(0.,0.,1.));
#9326=DIRECTION('',(1.,0.,0.));
#9327=DIRECTION('',(0.,0.,1.));
#9328=DIRECTION('center_axis',(0.,1.,0.));
#9329=DIRECTION('ref_axis',(0.,0.,1.));
#9330=DIRECTION('',(0.,0.,1.));
#9331=DIRECTION('',(1.,0.,0.));
#9332=DIRECTION('',(0.,0.,1.));
#9333=DIRECTION('center_axis',(0.,0.,-1.));
#9334=DIRECTION('ref_axis',(0.,1.,0.));
#9335=DIRECTION('',(0.,1.,0.));
#9336=DIRECTION('',(0.,1.,0.));
#9337=DIRECTION('center_axis',(0.,0.,-1.));
#9338=DIRECTION('ref_axis',(0.,1.,0.));
#9339=DIRECTION('',(0.,1.,0.));
#9340=DIRECTION('',(1.,0.,0.));
#9341=DIRECTION('',(0.,1.,0.));
#9342=DIRECTION('center_axis',(0.,-1.,0.));
#9343=DIRECTION('ref_axis',(0.,0.,-1.));
#9344=DIRECTION('',(0.,0.,-1.));
#9345=DIRECTION('',(0.,0.,-1.));
#9346=DIRECTION('center_axis',(0.,-1.,0.));
#9347=DIRECTION('ref_axis',(0.,0.,-1.));
#9348=DIRECTION('',(0.,0.,-1.));
#9349=DIRECTION('',(1.,0.,0.));
#9350=DIRECTION('',(0.,0.,-1.));
#9351=DIRECTION('center_axis',(0.,0.,1.));
#9352=DIRECTION('ref_axis',(0.,-1.,0.));
#9353=DIRECTION('',(0.,-1.,0.));
#9354=DIRECTION('',(0.,-1.,0.));
#9355=DIRECTION('center_axis',(0.,0.,1.));
#9356=DIRECTION('ref_axis',(0.,-1.,0.));
#9357=DIRECTION('',(0.,-1.,0.));
#9358=DIRECTION('',(0.,-1.,0.));
#9359=DIRECTION('center_axis',(1.,0.,0.));
#9360=DIRECTION('ref_axis',(0.,0.,-1.));
#9361=DIRECTION('center_axis',(1.,0.,0.));
#9362=DIRECTION('ref_axis',(0.,0.,-1.));
#11503=CARTESIAN_POINT('',(0.,0.,0.));
#11504=CARTESIAN_POINT('Origin',(14.,0.,-1.1));
#11505=CARTESIAN_POINT('',(13.725,-3.36777869765523E-17,-0.42));
#11506=CARTESIAN_POINT('Origin',(14.,0.,-0.42));
#11507=CARTESIAN_POINT('',(13.725,-4.28597456279282E-17,-0.21));
#11508=CARTESIAN_POINT('',(13.725,-3.36777869765523E-17,-1.1));
#11509=CARTESIAN_POINT('',(13.725,-1.33694465363225E-17,0.21));
#11510=CARTESIAN_POINT('Ctrl Pts',(13.725,2.60208521396521E-17,0.21));
#11511=CARTESIAN_POINT('Ctrl Pts',(13.725,-0.027663639322611,0.21));
#11512=CARTESIAN_POINT('Ctrl Pts',(13.7294937475236,-0.0563806217319969,
0.204214038345313));
#11513=CARTESIAN_POINT('Ctrl Pts',(13.7456015858723,-0.107860332287474,
0.182341144032027));
#11514=CARTESIAN_POINT('Ctrl Pts',(13.7571089410355,-0.130678518444188,
0.166306329654162));
#11515=CARTESIAN_POINT('Ctrl Pts',(13.7802392261772,-0.166732877511574,
0.130251970586776));
#11516=CARTESIAN_POINT('Ctrl Pts',(13.7937414503193,-0.182517999394844,
0.107475484252795));
#11517=CARTESIAN_POINT('Ctrl Pts',(13.8097472347118,-0.198712082533353,
0.0693141634661024));
#11518=CARTESIAN_POINT('Ctrl Pts',(13.8143361138528,-0.202908887997328,
0.0559106681449082));
#11519=CARTESIAN_POINT('Ctrl Pts',(13.8207009056693,-0.208554382393535,
0.0283388251429175));
#11520=CARTESIAN_POINT('Ctrl Pts',(13.8224471909544,-0.21,0.0141630178371274));
#11521=CARTESIAN_POINT('Ctrl Pts',(13.8224471909544,-0.21,-0.0141630178371274));
#11522=CARTESIAN_POINT('Ctrl Pts',(13.8207009056693,-0.208554382393535,
-0.0283388251429175));
#11523=CARTESIAN_POINT('Ctrl Pts',(13.8143361138528,-0.202908887997328,
-0.0559106681449082));
#11524=CARTESIAN_POINT('Ctrl Pts',(13.8097472347118,-0.198712082533353,
-0.0693141634661024));
#11525=CARTESIAN_POINT('Ctrl Pts',(13.7937414503193,-0.182517999394844,
-0.107475484252795));
#11526=CARTESIAN_POINT('Ctrl Pts',(13.7802392261772,-0.166732877511574,
-0.130251970586776));
#11527=CARTESIAN_POINT('Ctrl Pts',(13.7571089410355,-0.130678518444188,
-0.166306329654162));
#11528=CARTESIAN_POINT('Ctrl Pts',(13.7456015858723,-0.107860332287474,
-0.182341144032027));
#11529=CARTESIAN_POINT('Ctrl Pts',(13.7294937475236,-0.0563806217319969,
-0.204214038345313));
#11530=CARTESIAN_POINT('Ctrl Pts',(13.725,-0.0276636393226111,-0.21));
#11531=CARTESIAN_POINT('Ctrl Pts',(13.725,-3.81639164714898E-17,-0.21));
#11532=CARTESIAN_POINT('',(13.725,3.36777869765523E-17,0.42));
#11533=CARTESIAN_POINT('',(13.725,-3.36777869765523E-17,-1.1));
#11534=CARTESIAN_POINT('Origin',(14.,0.,0.42));
#11535=CARTESIAN_POINT('',(13.8224471909544,0.21,6.93889390390723E-18));
#11536=CARTESIAN_POINT('Ctrl Pts',(13.8224471909544,0.21,6.93889390390723E-18));
#11537=CARTESIAN_POINT('Ctrl Pts',(13.8224471909544,0.21,0.0141630178371274));
#11538=CARTESIAN_POINT('Ctrl Pts',(13.8207009056693,0.208554382393535,0.0283388251429175));
#11539=CARTESIAN_POINT('Ctrl Pts',(13.8143361138528,0.202908887997328,0.0559106681449082));
#11540=CARTESIAN_POINT('Ctrl Pts',(13.8097472347118,0.198712082533353,0.0693141634661024));
#11541=CARTESIAN_POINT('Ctrl Pts',(13.7937414503193,0.182517999394844,0.107475484252795));
#11542=CARTESIAN_POINT('Ctrl Pts',(13.7802392261772,0.166732877511574,0.130251970586776));
#11543=CARTESIAN_POINT('Ctrl Pts',(13.7571089410355,0.130678518444188,0.166306329654162));
#11544=CARTESIAN_POINT('Ctrl Pts',(13.7456015858723,0.107860332287474,0.182341144032027));
#11545=CARTESIAN_POINT('Ctrl Pts',(13.7294937475236,0.056380621731997,0.204214038345313));
#11546=CARTESIAN_POINT('Ctrl Pts',(13.725,0.0276636393226111,0.21));
#11547=CARTESIAN_POINT('Ctrl Pts',(13.725,2.60208521396521E-17,0.21));
#11548=CARTESIAN_POINT('Ctrl Pts',(13.725,-8.32667268468867E-17,-0.21));
#11549=CARTESIAN_POINT('Ctrl Pts',(13.725,0.0276636393226109,-0.21));
#11550=CARTESIAN_POINT('Ctrl Pts',(13.7294937475236,0.0563806217319968,
-0.204214038345313));
#11551=CARTESIAN_POINT('Ctrl Pts',(13.7456015858723,0.107860332287474,-0.182341144032027));
#11552=CARTESIAN_POINT('Ctrl Pts',(13.7571089410355,0.130678518444188,-0.166306329654162));
#11553=CARTESIAN_POINT('Ctrl Pts',(13.7802392261772,0.166732877511574,-0.130251970586776));
#11554=CARTESIAN_POINT('Ctrl Pts',(13.7937414503193,0.182517999394844,-0.107475484252795));
#11555=CARTESIAN_POINT('Ctrl Pts',(13.8097472347118,0.198712082533353,-0.0693141634661024));
#11556=CARTESIAN_POINT('Ctrl Pts',(13.8143361138528,0.202908887997328,-0.0559106681449082));
#11557=CARTESIAN_POINT('Ctrl Pts',(13.8207009056693,0.208554382393535,-0.0283388251429175));
#11558=CARTESIAN_POINT('Ctrl Pts',(13.8224471909544,0.21,-0.0141630178371274));
#11559=CARTESIAN_POINT('Ctrl Pts',(13.8224471909544,0.21,-4.85722573273506E-17));
#11560=CARTESIAN_POINT('',(14.1775528090456,0.21,5.89805981832114E-17));
#11561=CARTESIAN_POINT('',(14.275,4.48844336872086E-18,0.21));
#11562=CARTESIAN_POINT('Ctrl Pts',(14.1775528090456,0.21,5.89805981832114E-17));
#11563=CARTESIAN_POINT('Ctrl Pts',(14.1775528090456,0.21,-0.0141630178371273));
#11564=CARTESIAN_POINT('Ctrl Pts',(14.1792990943307,0.208554382393535,-0.0283388251429175));
#11565=CARTESIAN_POINT('Ctrl Pts',(14.1856638861472,0.202908887997328,-0.0559106681449082));
#11566=CARTESIAN_POINT('Ctrl Pts',(14.1902527652882,0.198712082533353,-0.0693141634661024));
#11567=CARTESIAN_POINT('Ctrl Pts',(14.2062585496807,0.182517999394844,-0.107475484252795));
#11568=CARTESIAN_POINT('Ctrl Pts',(14.2197607738228,0.166732877511574,-0.130251970586776));
#11569=CARTESIAN_POINT('Ctrl Pts',(14.2428910589645,0.130678518444188,-0.166306329654162));
#11570=CARTESIAN_POINT('Ctrl Pts',(14.2543984141277,0.107860332287473,-0.182341144032028));
#11571=CARTESIAN_POINT('Ctrl Pts',(14.2705062524764,0.056380621731996,-0.204214038345313));
#11572=CARTESIAN_POINT('Ctrl Pts',(14.275,0.027663639322611,-0.21));
#11573=CARTESIAN_POINT('Ctrl Pts',(14.275,-0.0276636393226111,-0.21));
#11574=CARTESIAN_POINT('Ctrl Pts',(14.2705062524764,-0.0563806217319969,
-0.204214038345313));
#11575=CARTESIAN_POINT('Ctrl Pts',(14.2543984141277,-0.107860332287474,
-0.182341144032027));
#11576=CARTESIAN_POINT('Ctrl Pts',(14.2428910589645,-0.130678518444188,
-0.166306329654162));
#11577=CARTESIAN_POINT('Ctrl Pts',(14.2197607738228,-0.166732877511574,
-0.130251970586776));
#11578=CARTESIAN_POINT('Ctrl Pts',(14.2062585496807,-0.182517999394844,
-0.107475484252795));
#11579=CARTESIAN_POINT('Ctrl Pts',(14.1902527652882,-0.198712082533353,
-0.0693141634661024));
#11580=CARTESIAN_POINT('Ctrl Pts',(14.1856638861472,-0.202908887997328,
-0.0559106681449082));
#11581=CARTESIAN_POINT('Ctrl Pts',(14.1792990943307,-0.208554382393535,
-0.0283388251429175));
#11582=CARTESIAN_POINT('Ctrl Pts',(14.1775528090456,-0.21,-0.0141630178371274));
#11583=CARTESIAN_POINT('Ctrl Pts',(14.1775528090456,-0.21,0.0141630178371274));
#11584=CARTESIAN_POINT('Ctrl Pts',(14.1792990943307,-0.208554382393535,
0.0283388251429175));
#11585=CARTESIAN_POINT('Ctrl Pts',(14.1856638861472,-0.202908887997328,
0.0559106681449082));
#11586=CARTESIAN_POINT('Ctrl Pts',(14.1902527652882,-0.198712082533353,
0.0693141634661024));
#11587=CARTESIAN_POINT('Ctrl Pts',(14.2062585496807,-0.182517999394844,
0.107475484252795));
#11588=CARTESIAN_POINT('Ctrl Pts',(14.2197607738228,-0.166732877511574,
0.130251970586776));
#11589=CARTESIAN_POINT('Ctrl Pts',(14.2428910589645,-0.130678518444188,
0.166306329654162));
#11590=CARTESIAN_POINT('Ctrl Pts',(14.2543984141277,-0.107860332287474,
0.182341144032027));
#11591=CARTESIAN_POINT('Ctrl Pts',(14.2705062524764,-0.056380621731997,
0.204214038345313));
#11592=CARTESIAN_POINT('Ctrl Pts',(14.275,-0.0276636393226111,0.21));
#11593=CARTESIAN_POINT('Ctrl Pts',(14.275,-3.81639164714898E-17,0.21));
#11594=CARTESIAN_POINT('Ctrl Pts',(14.275,1.38777878078145E-17,0.21));
#11595=CARTESIAN_POINT('Ctrl Pts',(14.275,0.027663639322611,0.21));
#11596=CARTESIAN_POINT('Ctrl Pts',(14.2705062524764,0.0563806217319969,
0.204214038345313));
#11597=CARTESIAN_POINT('Ctrl Pts',(14.2543984141277,0.107860332287474,0.182341144032027));
#11598=CARTESIAN_POINT('Ctrl Pts',(14.2428910589645,0.130678518444188,0.166306329654162));
#11599=CARTESIAN_POINT('Ctrl Pts',(14.2197607738228,0.166732877511574,0.130251970586776));
#11600=CARTESIAN_POINT('Ctrl Pts',(14.2062585496807,0.182517999394844,0.107475484252795));
#11601=CARTESIAN_POINT('Ctrl Pts',(14.1902527652882,0.198712082533353,0.0693141634661024));
#11602=CARTESIAN_POINT('Ctrl Pts',(14.1856638861472,0.202908887997328,0.0559106681449082));
#11603=CARTESIAN_POINT('Ctrl Pts',(14.1792990943307,0.208554382393535,0.0283388251429175));
#11604=CARTESIAN_POINT('Ctrl Pts',(14.1775528090456,0.21,0.0141630178371274));
#11605=CARTESIAN_POINT('Ctrl Pts',(14.1775528090456,0.21,-1.38777878078145E-17));
#11606=CARTESIAN_POINT('Origin',(-0.1,0.,0.));
#11607=CARTESIAN_POINT('',(0.,-2.57175827820944E-17,0.21));
#11608=CARTESIAN_POINT('Origin',(0.,0.,0.));
#11609=CARTESIAN_POINT('',(-0.1,-2.57175827820944E-17,0.21));
#11610=CARTESIAN_POINT('Origin',(-0.1,0.82,-0.3));
#11611=CARTESIAN_POINT('',(0.,0.82,-0.3));
#11612=CARTESIAN_POINT('',(0.,1.,-0.3));
#11613=CARTESIAN_POINT('',(0.,0.41,-0.3));
#11614=CARTESIAN_POINT('',(20.,0.82,-0.3));
#11615=CARTESIAN_POINT('',(-0.1,0.82,-0.3));
#11616=CARTESIAN_POINT('',(20.,1.,-0.3));
#11617=CARTESIAN_POINT('',(20.,0.41,-0.3));
#11618=CARTESIAN_POINT('',(-0.05,1.,-0.3));
#11619=CARTESIAN_POINT('Origin',(-0.1,0.82,-0.55));
#11620=CARTESIAN_POINT('',(0.,0.82,-0.55));
#11621=CARTESIAN_POINT('',(0.,0.82,-0.275));
#11622=CARTESIAN_POINT('',(20.,0.82,-0.55));
#11623=CARTESIAN_POINT('',(-0.1,0.82,-0.55));
#11624=CARTESIAN_POINT('',(20.,0.82,-0.275));
#11625=CARTESIAN_POINT('Origin',(-0.1,0.67,-0.55));
#11626=CARTESIAN_POINT('',(0.,0.67,-0.55));
#11627=CARTESIAN_POINT('',(0.,0.335,-0.55));
#11628=CARTESIAN_POINT('',(20.,0.67,-0.55));
#11629=CARTESIAN_POINT('',(-0.1,0.67,-0.55));
#11630=CARTESIAN_POINT('',(20.,0.335,-0.55));
#11631=CARTESIAN_POINT('Origin',(-0.1,0.42,-0.3));
#11632=CARTESIAN_POINT('',(0.,0.42,-0.3));
#11633=CARTESIAN_POINT('',(0.,0.24,-0.12));
#11634=CARTESIAN_POINT('',(20.,0.42,-0.3));
#11635=CARTESIAN_POINT('',(-0.1,0.42,-0.3));
#11636=CARTESIAN_POINT('',(20.,0.24,-0.12));
#11637=CARTESIAN_POINT('Origin',(-0.1,0.42,0.3));
#11638=CARTESIAN_POINT('',(0.,0.42,0.3));
#11639=CARTESIAN_POINT('',(0.,0.42,0.15));
#11640=CARTESIAN_POINT('',(20.,0.42,0.3));
#11641=CARTESIAN_POINT('',(-0.1,0.42,0.3));
#11642=CARTESIAN_POINT('',(20.,0.42,0.15));
#11643=CARTESIAN_POINT('Origin',(-0.1,0.67,0.55));
#11644=CARTESIAN_POINT('',(0.,0.67,0.55));
#11645=CARTESIAN_POINT('',(6.93889390390723E-18,0.365,0.245));
#11646=CARTESIAN_POINT('',(20.,0.67,0.55));
#11647=CARTESIAN_POINT('',(-0.1,0.67,0.55));
#11648=CARTESIAN_POINT('',(20.,0.365,0.245));
#11649=CARTESIAN_POINT('Origin',(-0.1,0.82,0.55));
#11650=CARTESIAN_POINT('',(0.,0.82,0.55));
#11651=CARTESIAN_POINT('',(0.,0.41,0.55));
#11652=CARTESIAN_POINT('',(20.,0.82,0.55));
#11653=CARTESIAN_POINT('',(-0.1,0.82,0.55));
#11654=CARTESIAN_POINT('',(20.,0.41,0.55));
#11655=CARTESIAN_POINT('Origin',(-0.1,0.82,0.3));
#11656=CARTESIAN_POINT('',(0.,0.82,0.3));
#11657=CARTESIAN_POINT('',(0.,0.82,0.15));
#11658=CARTESIAN_POINT('',(20.,0.82,0.3));
#11659=CARTESIAN_POINT('',(-0.1,0.82,0.3));
#11660=CARTESIAN_POINT('',(20.,0.82,0.15));
#11661=CARTESIAN_POINT('Origin',(-0.1,1.05,0.3));
#11662=CARTESIAN_POINT('',(0.,1.,0.3));
#11663=CARTESIAN_POINT('',(0.,0.525,0.3));
#11664=CARTESIAN_POINT('',(20.,1.,0.3));
#11665=CARTESIAN_POINT('',(-0.05,1.,0.3));
#11666=CARTESIAN_POINT('',(20.,0.525,0.3));
#11667=CARTESIAN_POINT('Origin',(-0.1,-0.3,-0.82));
#11668=CARTESIAN_POINT('',(0.,-0.3,-0.82));
#11669=CARTESIAN_POINT('',(0.,-0.3,-1.));
#11670=CARTESIAN_POINT('',(0.,-0.3,-0.41));
#11671=CARTESIAN_POINT('',(20.,-0.3,-0.82));
#11672=CARTESIAN_POINT('',(-0.1,-0.3,-0.82));
#11673=CARTESIAN_POINT('',(20.,-0.3,-1.));
#11674=CARTESIAN_POINT('',(20.,-0.3,-0.41));
#11675=CARTESIAN_POINT('',(-0.05,-0.3,-1.));
#11676=CARTESIAN_POINT('Origin',(-0.1,-0.55,-0.82));
#11677=CARTESIAN_POINT('',(0.,-0.55,-0.82));
#11678=CARTESIAN_POINT('',(0.,-0.275,-0.82));
#11679=CARTESIAN_POINT('',(20.,-0.55,-0.82));
#11680=CARTESIAN_POINT('',(-0.1,-0.55,-0.82));
#11681=CARTESIAN_POINT('',(20.,-0.275,-0.82));
#11682=CARTESIAN_POINT('Origin',(-0.1,-0.55,-0.67));
#11683=CARTESIAN_POINT('',(0.,-0.55,-0.67));
#11684=CARTESIAN_POINT('',(0.,-0.55,-0.335));
#11685=CARTESIAN_POINT('',(20.,-0.55,-0.67));
#11686=CARTESIAN_POINT('',(-0.1,-0.55,-0.67));
#11687=CARTESIAN_POINT('',(20.,-0.55,-0.335));
#11688=CARTESIAN_POINT('Origin',(-0.1,-0.3,-0.42));
#11689=CARTESIAN_POINT('',(0.,-0.3,-0.42));
#11690=CARTESIAN_POINT('',(0.,-0.12,-0.24));
#11691=CARTESIAN_POINT('',(20.,-0.3,-0.42));
#11692=CARTESIAN_POINT('',(-0.1,-0.3,-0.42));
#11693=CARTESIAN_POINT('',(20.,-0.12,-0.24));
#11694=CARTESIAN_POINT('Origin',(-0.1,0.3,-0.42));
#11695=CARTESIAN_POINT('',(0.,0.3,-0.42));
#11696=CARTESIAN_POINT('',(0.,0.15,-0.42));
#11697=CARTESIAN_POINT('',(20.,0.3,-0.42));
#11698=CARTESIAN_POINT('',(-0.1,0.3,-0.42));
#11699=CARTESIAN_POINT('',(20.,0.15,-0.42));
#11700=CARTESIAN_POINT('Origin',(-0.1,0.55,-0.67));
#11701=CARTESIAN_POINT('',(0.,0.55,-0.67));
#11702=CARTESIAN_POINT('',(0.,0.245,-0.365));
#11703=CARTESIAN_POINT('',(20.,0.55,-0.67));
#11704=CARTESIAN_POINT('',(-0.1,0.55,-0.67));
#11705=CARTESIAN_POINT('',(20.,0.245,-0.365));
#11706=CARTESIAN_POINT('Origin',(-0.1,0.55,-0.82));
#11707=CARTESIAN_POINT('',(0.,0.55,-0.82));
#11708=CARTESIAN_POINT('',(0.,0.55,-0.41));
#11709=CARTESIAN_POINT('',(20.,0.55,-0.82));
#11710=CARTESIAN_POINT('',(-0.1,0.55,-0.82));
#11711=CARTESIAN_POINT('',(20.,0.55,-0.41));
#11712=CARTESIAN_POINT('Origin',(-0.1,0.3,-0.82));
#11713=CARTESIAN_POINT('',(0.,0.3,-0.82));
#11714=CARTESIAN_POINT('',(0.,0.15,-0.82));
#11715=CARTESIAN_POINT('',(20.,0.3,-0.82));
#11716=CARTESIAN_POINT('',(-0.1,0.3,-0.82));
#11717=CARTESIAN_POINT('',(20.,0.15,-0.82));
#11718=CARTESIAN_POINT('Origin',(-0.1,0.3,-1.05));
#11719=CARTESIAN_POINT('',(0.,0.3,-1.));
#11720=CARTESIAN_POINT('',(0.,0.3,-0.525));
#11721=CARTESIAN_POINT('',(20.,0.3,-1.));
#11722=CARTESIAN_POINT('',(-0.05,0.3,-1.));
#11723=CARTESIAN_POINT('',(20.,0.3,-0.525));
#11724=CARTESIAN_POINT('Origin',(-0.1,-0.82,0.3));
#11725=CARTESIAN_POINT('',(0.,-0.82,0.3));
#11726=CARTESIAN_POINT('',(0.,-1.,0.3));
#11727=CARTESIAN_POINT('',(0.,-0.41,0.3));
#11728=CARTESIAN_POINT('',(20.,-0.82,0.3));
#11729=CARTESIAN_POINT('',(-0.1,-0.82,0.3));
#11730=CARTESIAN_POINT('',(20.,-1.,0.3));
#11731=CARTESIAN_POINT('',(20.,-0.41,0.3));
#11732=CARTESIAN_POINT('',(-0.05,-1.,0.3));
#11733=CARTESIAN_POINT('Origin',(-0.1,-0.82,0.55));
#11734=CARTESIAN_POINT('',(0.,-0.82,0.55));
#11735=CARTESIAN_POINT('',(0.,-0.82,0.275));
#11736=CARTESIAN_POINT('',(20.,-0.82,0.55));
#11737=CARTESIAN_POINT('',(-0.1,-0.82,0.55));
#11738=CARTESIAN_POINT('',(20.,-0.82,0.275));
#11739=CARTESIAN_POINT('Origin',(-0.1,-0.67,0.55));
#11740=CARTESIAN_POINT('',(0.,-0.67,0.55));
#11741=CARTESIAN_POINT('',(0.,-0.335,0.55));
#11742=CARTESIAN_POINT('',(20.,-0.67,0.55));
#11743=CARTESIAN_POINT('',(-0.1,-0.67,0.55));
#11744=CARTESIAN_POINT('',(20.,-0.335,0.55));
#11745=CARTESIAN_POINT('Origin',(-0.1,-0.42,0.3));
#11746=CARTESIAN_POINT('',(0.,-0.42,0.3));
#11747=CARTESIAN_POINT('',(-6.93889390390723E-18,-0.24,0.12));
#11748=CARTESIAN_POINT('',(20.,-0.42,0.3));
#11749=CARTESIAN_POINT('',(-0.1,-0.42,0.3));
#11750=CARTESIAN_POINT('',(20.,-0.24,0.12));
#11751=CARTESIAN_POINT('Origin',(-0.1,-0.42,-0.3));
#11752=CARTESIAN_POINT('',(0.,-0.42,-0.3));
#11753=CARTESIAN_POINT('',(0.,-0.42,-0.15));
#11754=CARTESIAN_POINT('',(20.,-0.42,-0.3));
#11755=CARTESIAN_POINT('',(-0.1,-0.42,-0.3));
#11756=CARTESIAN_POINT('',(20.,-0.42,-0.15));
#11757=CARTESIAN_POINT('Origin',(-0.1,-0.67,-0.55));
#11758=CARTESIAN_POINT('',(0.,-0.67,-0.55));
#11759=CARTESIAN_POINT('',(0.,-0.365,-0.245));
#11760=CARTESIAN_POINT('',(20.,-0.67,-0.55));
#11761=CARTESIAN_POINT('',(-0.1,-0.67,-0.55));
#11762=CARTESIAN_POINT('',(20.,-0.365,-0.245));
#11763=CARTESIAN_POINT('Origin',(-0.1,-0.82,-0.55));
#11764=CARTESIAN_POINT('',(0.,-0.82,-0.55));
#11765=CARTESIAN_POINT('',(0.,-0.41,-0.55));
#11766=CARTESIAN_POINT('',(20.,-0.82,-0.55));
#11767=CARTESIAN_POINT('',(-0.1,-0.82,-0.55));
#11768=CARTESIAN_POINT('',(20.,-0.41,-0.55));
#11769=CARTESIAN_POINT('Origin',(-0.1,-0.82,-0.3));
#11770=CARTESIAN_POINT('',(0.,-0.82,-0.3));
#11771=CARTESIAN_POINT('',(0.,-0.82,-0.15));
#11772=CARTESIAN_POINT('',(20.,-0.82,-0.3));
#11773=CARTESIAN_POINT('',(-0.1,-0.82,-0.3));
#11774=CARTESIAN_POINT('',(20.,-0.82,-0.15));
#11775=CARTESIAN_POINT('Origin',(-0.1,-1.05,-0.3));
#11776=CARTESIAN_POINT('',(0.,-1.,-0.3));
#11777=CARTESIAN_POINT('',(0.,-0.525,-0.3));
#11778=CARTESIAN_POINT('',(20.,-1.,-0.3));
#11779=CARTESIAN_POINT('',(-0.05,-1.,-0.3));
#11780=CARTESIAN_POINT('',(20.,-0.525,-0.3));
#11781=CARTESIAN_POINT('Origin',(-0.1,0.3,0.82));
#11782=CARTESIAN_POINT('',(0.,0.3,0.82));
#11783=CARTESIAN_POINT('',(0.,0.3,1.));
#11784=CARTESIAN_POINT('',(0.,0.3,0.41));
#11785=CARTESIAN_POINT('',(20.,0.3,0.82));
#11786=CARTESIAN_POINT('',(-0.1,0.3,0.82));
#11787=CARTESIAN_POINT('',(20.,0.3,1.));
#11788=CARTESIAN_POINT('',(20.,0.3,0.41));
#11789=CARTESIAN_POINT('',(-0.05,0.3,1.));
#11790=CARTESIAN_POINT('Origin',(-0.1,0.55,0.82));
#11791=CARTESIAN_POINT('',(0.,0.55,0.82));
#11792=CARTESIAN_POINT('',(0.,0.275,0.82));
#11793=CARTESIAN_POINT('',(20.,0.55,0.82));
#11794=CARTESIAN_POINT('',(-0.1,0.55,0.82));
#11795=CARTESIAN_POINT('',(20.,0.275,0.82));
#11796=CARTESIAN_POINT('Origin',(-0.1,0.55,0.67));
#11797=CARTESIAN_POINT('',(0.,0.55,0.67));
#11798=CARTESIAN_POINT('',(0.,0.55,0.335));
#11799=CARTESIAN_POINT('',(20.,0.55,0.67));
#11800=CARTESIAN_POINT('',(-0.1,0.55,0.67));
#11801=CARTESIAN_POINT('',(20.,0.55,0.335));
#11802=CARTESIAN_POINT('Origin',(-0.1,0.3,0.42));
#11803=CARTESIAN_POINT('',(0.,0.3,0.42));
#11804=CARTESIAN_POINT('',(6.93889390390723E-18,0.12,0.24));
#11805=CARTESIAN_POINT('',(20.,0.3,0.42));
#11806=CARTESIAN_POINT('',(-0.1,0.3,0.42));
#11807=CARTESIAN_POINT('',(20.,0.12,0.24));
#11808=CARTESIAN_POINT('Origin',(-0.1,-0.3,0.42));
#11809=CARTESIAN_POINT('',(0.,-0.3,0.42));
#11810=CARTESIAN_POINT('',(0.,-0.15,0.42));
#11811=CARTESIAN_POINT('',(20.,-0.3,0.42));
#11812=CARTESIAN_POINT('',(-0.1,-0.3,0.42));
#11813=CARTESIAN_POINT('',(20.,-0.15,0.42));
#11814=CARTESIAN_POINT('Origin',(-0.1,-0.55,0.67));
#11815=CARTESIAN_POINT('',(0.,-0.55,0.67));
#11816=CARTESIAN_POINT('',(6.93889390390723E-18,-0.245,0.365));
#11817=CARTESIAN_POINT('',(20.,-0.55,0.67));
#11818=CARTESIAN_POINT('',(-0.1,-0.55,0.67));
#11819=CARTESIAN_POINT('',(20.,-0.245,0.365));
#11820=CARTESIAN_POINT('Origin',(-0.1,-0.55,0.82));
#11821=CARTESIAN_POINT('',(0.,-0.55,0.82));
#11822=CARTESIAN_POINT('',(0.,-0.55,0.41));
#11823=CARTESIAN_POINT('',(20.,-0.55,0.82));
#11824=CARTESIAN_POINT('',(-0.1,-0.55,0.82));
#11825=CARTESIAN_POINT('',(20.,-0.55,0.41));
#11826=CARTESIAN_POINT('Origin',(-0.1,-0.3,0.82));
#11827=CARTESIAN_POINT('',(0.,-0.3,0.82));
#11828=CARTESIAN_POINT('',(0.,-0.15,0.82));
#11829=CARTESIAN_POINT('',(20.,-0.3,0.82));
#11830=CARTESIAN_POINT('',(-0.1,-0.3,0.82));
#11831=CARTESIAN_POINT('',(20.,-0.15,0.82));
#11832=CARTESIAN_POINT('Origin',(-0.1,-0.3,1.05));
#11833=CARTESIAN_POINT('',(0.,-0.3,1.));
#11834=CARTESIAN_POINT('',(0.,-0.3,0.525));
#11835=CARTESIAN_POINT('',(20.,-0.3,1.));
#11836=CARTESIAN_POINT('',(-0.05,-0.3,1.));
#11837=CARTESIAN_POINT('',(20.,-0.3,0.525));
#11838=CARTESIAN_POINT('Origin',(-0.1,0.,0.));
#11839=CARTESIAN_POINT('',(20.,2.57175827820944E-17,0.21));
#11840=CARTESIAN_POINT('',(-0.1,-2.57175827820944E-17,0.21));
#11841=CARTESIAN_POINT('Origin',(20.,0.,0.));
#11842=CARTESIAN_POINT('Origin',(0.,1.,-1.));
#11843=CARTESIAN_POINT('',(0.,1.,1.));
#11844=CARTESIAN_POINT('',(0.,1.,-1.));
#11845=CARTESIAN_POINT('',(20.,1.,1.));
#11846=CARTESIAN_POINT('',(0.,1.,1.));
#11847=CARTESIAN_POINT('',(20.,1.,-1.));
#11848=CARTESIAN_POINT('Origin',(0.,1.,-1.));
#11849=CARTESIAN_POINT('',(20.,1.,-1.));
#11850=CARTESIAN_POINT('',(20.,1.,-1.));
#11851=CARTESIAN_POINT('',(0.,1.,-1.));
#11852=CARTESIAN_POINT('',(0.,1.,-1.));
#11853=CARTESIAN_POINT('',(0.,1.,-1.));
#11854=CARTESIAN_POINT('Origin',(0.,-1.,-1.));
#11855=CARTESIAN_POINT('',(0.,-1.,-1.));
#11856=CARTESIAN_POINT('',(20.,-1.,-1.));
#11857=CARTESIAN_POINT('Origin',(0.,-1.,-1.));
#11858=CARTESIAN_POINT('',(20.,-1.,-1.));
#11859=CARTESIAN_POINT('',(20.,-1.,-1.));
#11860=CARTESIAN_POINT('',(0.,-1.,-1.));
#11861=CARTESIAN_POINT('',(0.,-1.,-1.));
#11862=CARTESIAN_POINT('',(0.,-1.,-1.));
#11863=CARTESIAN_POINT('Origin',(0.,-1.,1.));
#11864=CARTESIAN_POINT('',(0.,-1.,1.));
#11865=CARTESIAN_POINT('',(20.,-1.,1.));
#11866=CARTESIAN_POINT('Origin',(0.,-1.,1.));
#11867=CARTESIAN_POINT('',(20.,-1.,1.));
#11868=CARTESIAN_POINT('',(20.,-1.,1.));
#11869=CARTESIAN_POINT('',(0.,-1.,1.));
#11870=CARTESIAN_POINT('',(0.,-1.,1.));
#11871=CARTESIAN_POINT('',(0.,-1.,1.));
#11872=CARTESIAN_POINT('Origin',(0.,1.,1.));
#11873=CARTESIAN_POINT('',(0.,1.,1.));
#11874=CARTESIAN_POINT('',(20.,1.,1.));
#11875=CARTESIAN_POINT('Origin',(0.,1.,1.));
#11876=CARTESIAN_POINT('',(20.,1.,1.));
#11877=CARTESIAN_POINT('',(0.,1.,1.));
#11878=CARTESIAN_POINT('Origin',(20.,0.,0.));
#11879=CARTESIAN_POINT('Origin',(0.,0.,0.));
#13748=UNCERTAINTY_MEASURE_WITH_UNIT(LENGTH_MEASURE(0.001),#13822,
'DISTANCE_ACCURACY_VALUE',
'Maximum model space distance between geometric entities at asserted c
onnectivities');
#13782=UNCERTAINTY_MEASURE_WITH_UNIT(LENGTH_MEASURE(0.001),#13822,
'DISTANCE_ACCURACY_VALUE',
'Maximum model space distance between geometric entities at asserted c
onnectivities');
#13787=(
GEOMETRIC_REPRESENTATION_CONTEXT(3)
GLOBAL_UNCERTAINTY_ASSIGNED_CONTEXT((#13748))
GLOBAL_UNIT_ASSIGNED_CONTEXT((#13822,#13824,#13825))
REPRESENTATION_CONTEXT('','3D')
);
#13821=(
GEOMETRIC_REPRESENTATION_CONTEXT(3)
GLOBAL_UNCERTAINTY_ASSIGNED_CONTEXT((#13782))
GLOBAL_UNIT_ASSIGNED_CONTEXT((#13822,#13824,#13825))
REPRESENTATION_CONTEXT('','3D')
);
#13822=(
LENGTH_UNIT()
NAMED_UNIT(*)
SI_UNIT(.CENTI.,.METRE.)
);
#13824=(
NAMED_UNIT(*)
PLANE_ANGLE_UNIT()
SI_UNIT($,.RADIAN.)
);
#13825=(
NAMED_UNIT(*)
SI_UNIT($,.STERADIAN.)
SOLID_ANGLE_UNIT()
);
#13830=SHAPE_DEFINITION_REPRESENTATION(#13868,#14000);
#13868=PRODUCT_DEFINITION_SHAPE('',$,#14039);
#14000=SHAPE_REPRESENTATION('',(#8123),#13787);
#14034=PRODUCT_DEFINITION_CONTEXT('part definition',#14150,'design');
#14039=PRODUCT_DEFINITION('Drilled 200 mm rail','Drilled 200 mm rail',#14077,
#14034);
#14077=PRODUCT_DEFINITION_FORMATION('',$,#14156);
#14150=APPLICATION_CONTEXT(
'Core Data for Automotive Mechanical Design Process');
#14151=PRODUCT_CONTEXT('part definition',#14150,'mechanical');
#14156=PRODUCT('Drilled 200 mm rail','Drilled 200 mm rail',
'Drilled 200 mm rail',(#14151));
#14191=PRESENTATION_STYLE_ASSIGNMENT((#14196));
#14196=SURFACE_STYLE_USAGE(.BOTH.,#14201);
#14201=SURFACE_SIDE_STYLE('',(#14206));
#14206=SURFACE_STYLE_FILL_AREA(#14211);
#14211=FILL_AREA_STYLE('CAD Library Painted - Steel gray',(#14216));
#14216=FILL_AREA_STYLE_COLOUR('CAD Library Painted - Steel gray',#14221);
#14221=COLOUR_RGB('CAD Library Painted - Steel gray',0.592156862745098,
0.631372549019608,0.67843137254902);
ENDSEC;
END-ISO-10303-21;
